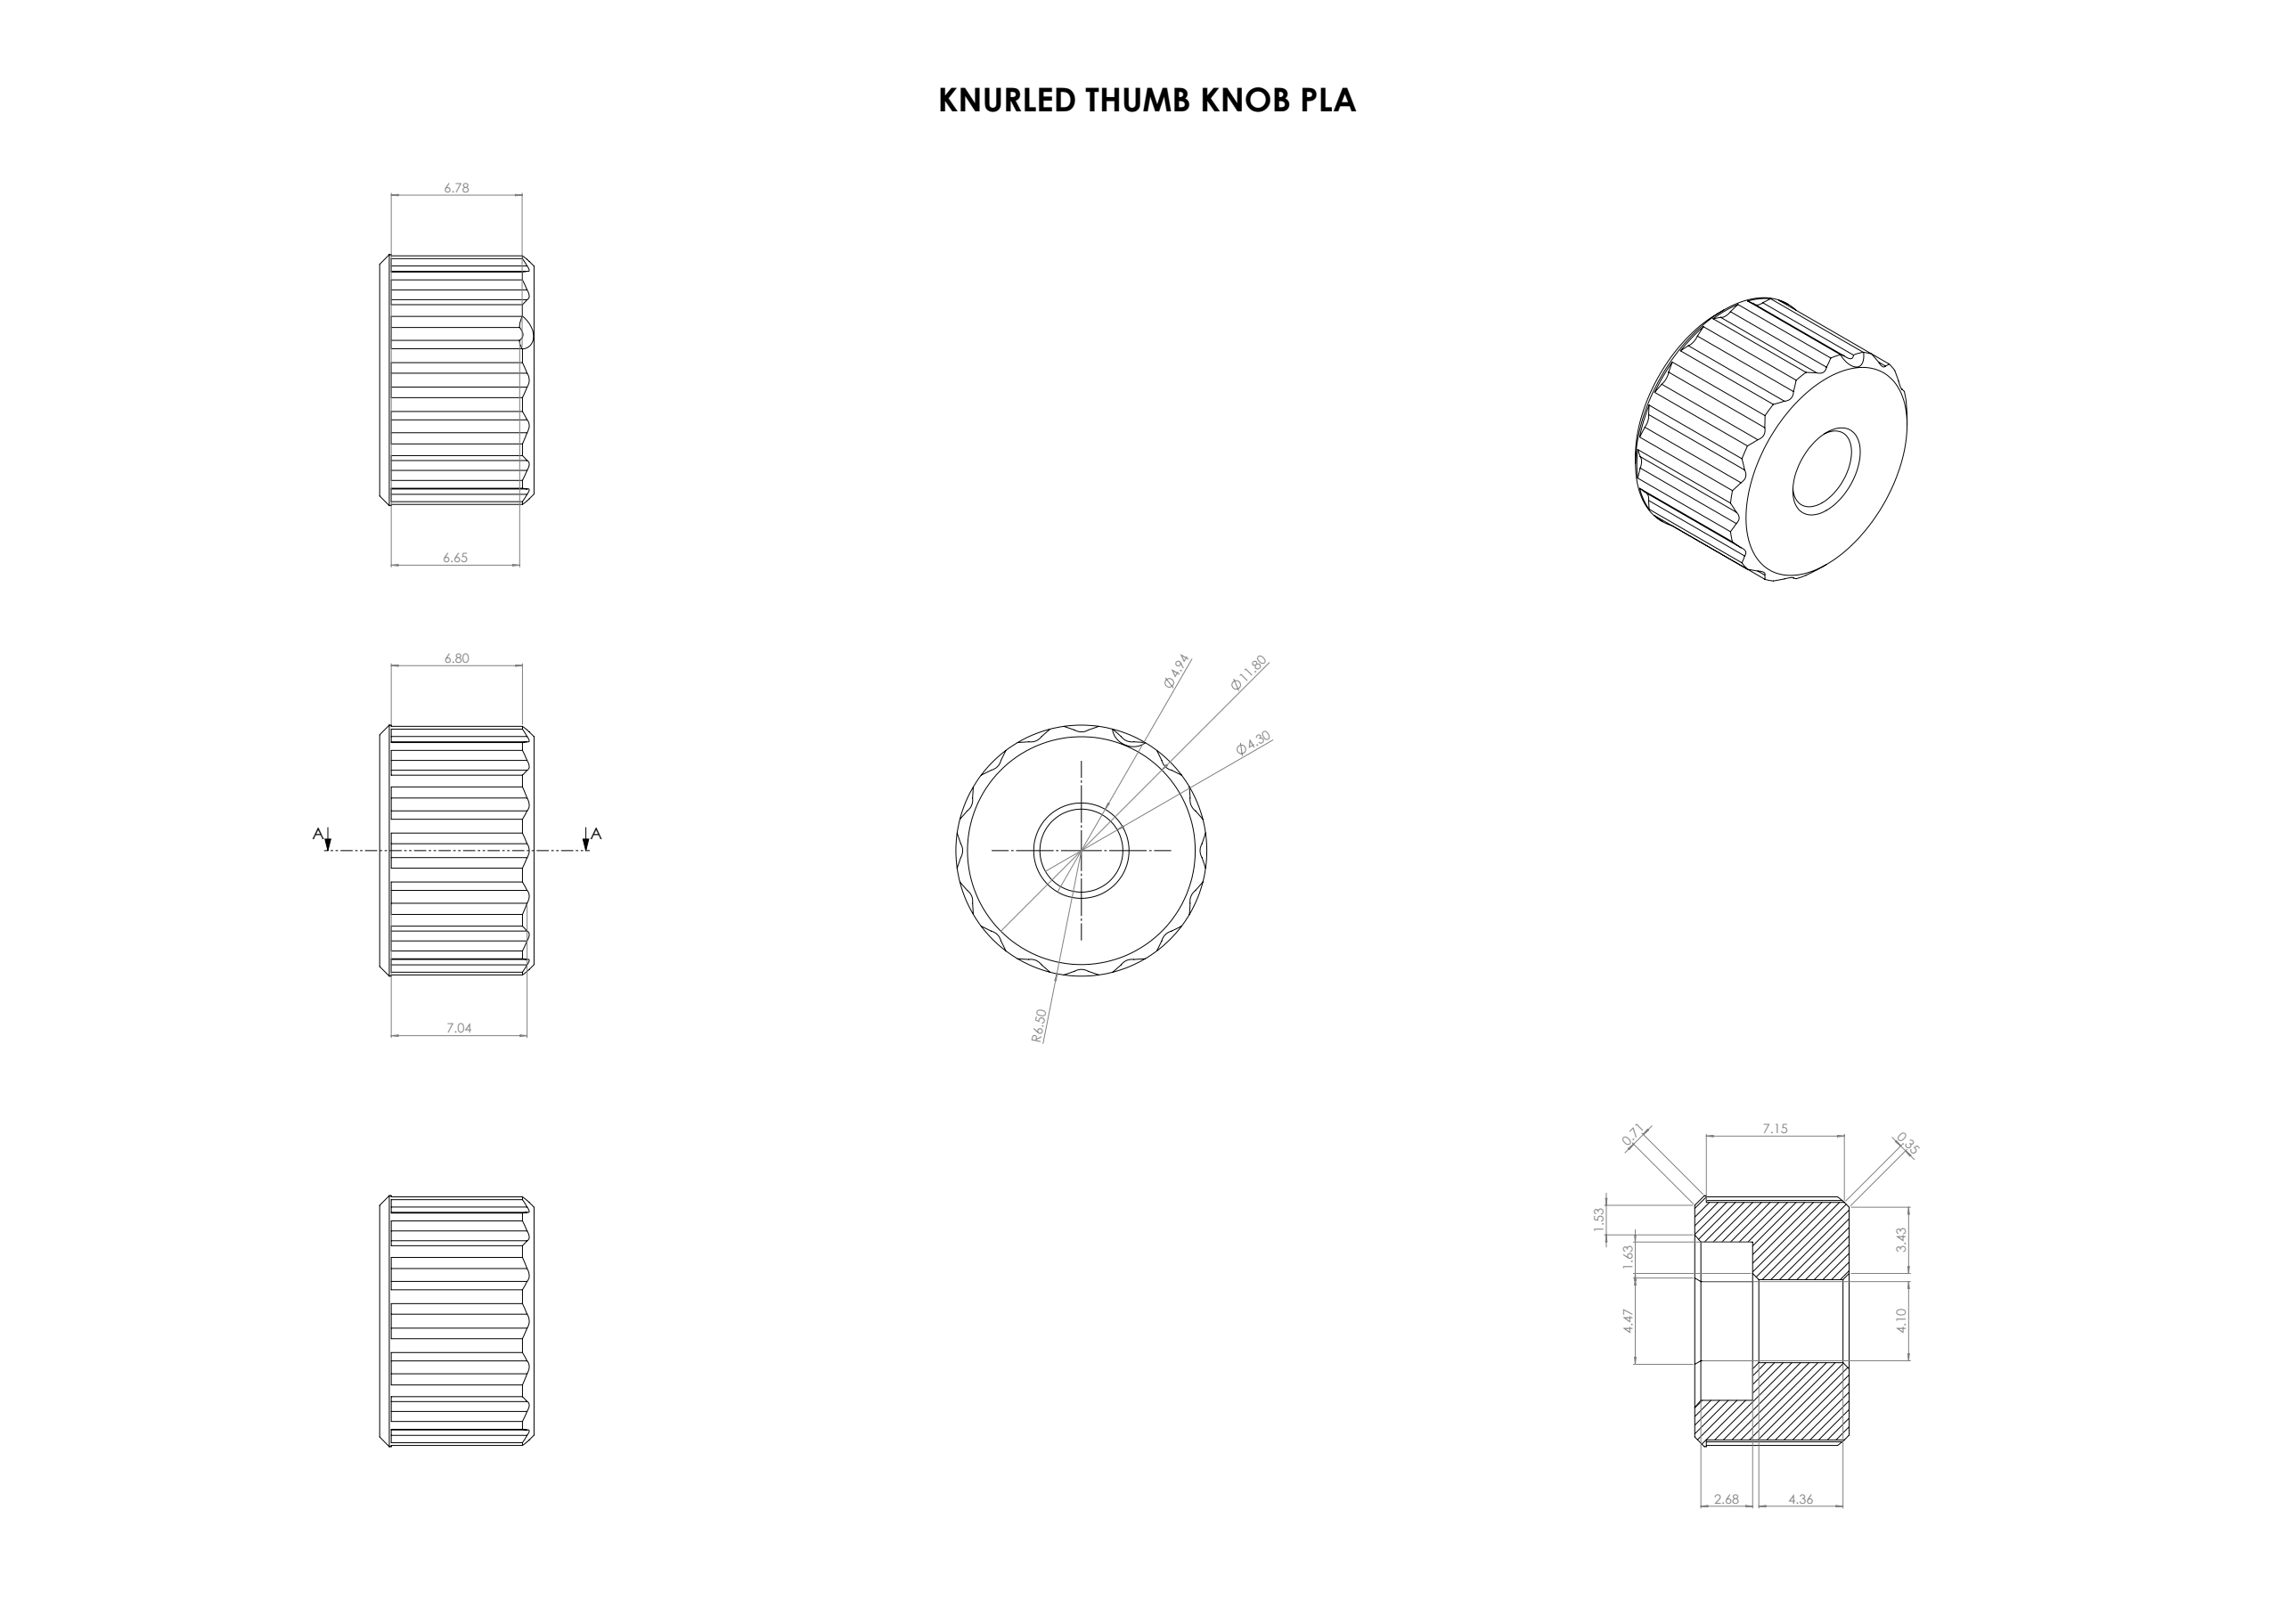
ISO-10303-21;
HEADER;
/* Generated by software containing ST-Developer
 * from STEP Tools, Inc. (www.steptools.com) 
 */

FILE_DESCRIPTION(
/* description */ (''),
/* implementation_level */ '2;1');

FILE_NAME(
/* name */ '08_Knurled_Thumb_Knob_PLA.step',
/* time_stamp */ '2026-10-21T02:01:14-07:00',
/* author */ (''),
/* organization */ (''),
/* preprocessor_version */ 'ST-DEVELOPER v20.2',
/* originating_system */ 'Autodesk Translation Framework v15.15.0.0',
/* authorisation */ '');

FILE_SCHEMA (('AUTOMOTIVE_DESIGN { 1 0 10303 214 3 1 1 }'));
ENDSEC;

DATA;
#10=MECHANICAL_DESIGN_GEOMETRIC_PRESENTATION_REPRESENTATION('',(#621),#37181);
#113=B_SPLINE_SURFACE_WITH_KNOTS('',3,3,((#26771,#26772,#26773,#26774,#26775,
#26776,#26777,#26778,#26779),(#26780,#26781,#26782,#26783,#26784,#26785,
#26786,#26787,#26788),(#26789,#26790,#26791,#26792,#26793,#26794,#26795,
#26796,#26797),(#26798,#26799,#26800,#26801,#26802,#26803,#26804,#26805,
#26806)),.UNSPECIFIED.,.F.,.F.,.F.,(4,4),(4,1,1,1,1,1,4),(0.,1.),(0.0342009647377285,
0.0587640238978664,0.0833270830580044,0.107890142218142,0.13245320137828,
0.181579319698556,0.206142378858694),.UNSPECIFIED.);
#259=B_SPLINE_CURVE_WITH_KNOTS('',3,(#26240,#26241,#26242,#26243),
 .UNSPECIFIED.,.F.,.F.,(4,4),(0.0531689808046697,0.0554215660138355),
 .UNSPECIFIED.);
#260=B_SPLINE_CURVE_WITH_KNOTS('',3,(#26251,#26252,#26253,#26254),
 .UNSPECIFIED.,.F.,.F.,(4,4),(0.,0.00224311679852086),.UNSPECIFIED.);
#261=B_SPLINE_CURVE_WITH_KNOTS('',3,(#26379,#26380,#26381,#26382,#26383,
#26384),.UNSPECIFIED.,.F.,.F.,(4,2,4),(0.120171671798206,0.144386237549695,
0.158573008898185),.UNSPECIFIED.);
#262=B_SPLINE_CURVE_WITH_KNOTS('',3,(#26393,#26394,#26395,#26396,#26397,
#26398,#26399,#26400,#26401,#26402),.UNSPECIFIED.,.F.,.F.,(4,2,2,2,4),(0.0817703346982273,
0.0959571060467179,0.120171671798206,0.144386237549695,0.158573008898185),
 .UNSPECIFIED.);
#263=B_SPLINE_CURVE_WITH_KNOTS('',3,(#26411,#26412,#26413,#26414,#26415,
#26416,#26417,#26418,#26419,#26420),.UNSPECIFIED.,.F.,.F.,(4,2,2,2,4),(0.0817703346982278,
0.095957106046718,0.120171671798206,0.144386237549695,0.158573008898185),
 .UNSPECIFIED.);
#264=B_SPLINE_CURVE_WITH_KNOTS('',3,(#26429,#26430,#26431,#26432,#26433,
#26434,#26435,#26436,#26437,#26438),.UNSPECIFIED.,.F.,.F.,(4,2,2,2,4),(0.0817703346982272,
0.0959571060467179,0.120171671798206,0.144386237549695,0.158573008898185),
 .UNSPECIFIED.);
#265=B_SPLINE_CURVE_WITH_KNOTS('',3,(#26447,#26448,#26449,#26450,#26451,
#26452,#26453,#26454,#26455,#26456),.UNSPECIFIED.,.F.,.F.,(4,2,2,2,4),(0.0817703346982273,
0.0959571060467178,0.120171671798206,0.144386237549695,0.158573008898185),
 .UNSPECIFIED.);
#266=B_SPLINE_CURVE_WITH_KNOTS('',3,(#26465,#26466,#26467,#26468,#26469,
#26470,#26471,#26472,#26473,#26474),.UNSPECIFIED.,.F.,.F.,(4,2,2,2,4),(0.081770334698227,
0.0959571060467179,0.120171671798206,0.144386237549695,0.158573008898185),
 .UNSPECIFIED.);
#267=B_SPLINE_CURVE_WITH_KNOTS('',3,(#26483,#26484,#26485,#26486,#26487,
#26488,#26489,#26490,#26491,#26492),.UNSPECIFIED.,.F.,.F.,(4,2,2,2,4),(0.0817703346982273,
0.0959571060467179,0.120171671798206,0.144386237549695,0.158573008898185),
 .UNSPECIFIED.);
#268=B_SPLINE_CURVE_WITH_KNOTS('',3,(#26496,#26497,#26498,#26499,#26500,
#26501,#26502,#26503,#26504),.UNSPECIFIED.,.F.,.F.,(4,1,1,1,1,1,4),(-0.20552137705515,
-0.181579319698556,-0.13245320137828,-0.107890142218142,-0.0833270830580044,
-0.0587640238978664,-0.0348207934698036),.UNSPECIFIED.);
#269=B_SPLINE_CURVE_WITH_KNOTS('',3,(#26506,#26507,#26508,#26509,#26510,
#26511,#26512,#26513,#26514,#26515),.UNSPECIFIED.,.F.,.F.,(4,2,2,2,4),(0.0817703346982273,
0.0959571060467179,0.120171671798206,0.144386237549695,0.158573008898185),
 .UNSPECIFIED.);
#270=B_SPLINE_CURVE_WITH_KNOTS('',3,(#26524,#26525,#26526,#26527,#26528,
#26529,#26530,#26531,#26532,#26533),.UNSPECIFIED.,.F.,.F.,(4,2,2,2,4),(0.0817703346982272,
0.095957106046718,0.120171671798206,0.144386237549695,0.158573008898185),
 .UNSPECIFIED.);
#271=B_SPLINE_CURVE_WITH_KNOTS('',3,(#26542,#26543,#26544,#26545,#26546,
#26547,#26548,#26549,#26550,#26551),.UNSPECIFIED.,.F.,.F.,(4,2,2,2,4),(0.0817703346982275,
0.095957106046718,0.120171671798206,0.144386237549695,0.158573008898185),
 .UNSPECIFIED.);
#272=B_SPLINE_CURVE_WITH_KNOTS('',3,(#26560,#26561,#26562,#26563,#26564,
#26565,#26566,#26567,#26568,#26569),.UNSPECIFIED.,.F.,.F.,(4,2,2,2,4),(0.0817703346982276,
0.095957106046718,0.120171671798206,0.144386237549695,0.158573008898185),
 .UNSPECIFIED.);
#273=B_SPLINE_CURVE_WITH_KNOTS('',3,(#26578,#26579,#26580,#26581,#26582,
#26583,#26584,#26585,#26586,#26587),.UNSPECIFIED.,.F.,.F.,(4,2,2,2,4),(0.0817703346982272,
0.0959571060467178,0.120171671798206,0.144386237549695,0.158573008898185),
 .UNSPECIFIED.);
#274=B_SPLINE_CURVE_WITH_KNOTS('',3,(#26596,#26597,#26598,#26599,#26600,
#26601,#26602,#26603,#26604,#26605),.UNSPECIFIED.,.F.,.F.,(4,2,2,2,4),(0.0817703346982273,
0.0959571060467179,0.120171671798206,0.144386237549695,0.158573008898185),
 .UNSPECIFIED.);
#275=B_SPLINE_CURVE_WITH_KNOTS('',3,(#26614,#26615,#26616,#26617,#26618,
#26619,#26620,#26621,#26622,#26623),.UNSPECIFIED.,.F.,.F.,(4,2,2,2,4),(0.0817703346982272,
0.0959571060467179,0.120171671798206,0.144386237549695,0.158573008898185),
 .UNSPECIFIED.);
#276=B_SPLINE_CURVE_WITH_KNOTS('',3,(#26632,#26633,#26634,#26635,#26636,
#26637,#26638,#26639,#26640,#26641),.UNSPECIFIED.,.F.,.F.,(4,2,2,2,4),(0.0817703346982276,
0.095957106046718,0.120171671798206,0.144386237549695,0.158573008898185),
 .UNSPECIFIED.);
#277=B_SPLINE_CURVE_WITH_KNOTS('',3,(#26649,#26650,#26651,#26652,#26653,
#26654),.UNSPECIFIED.,.F.,.F.,(4,2,4),(0.0817703346982272,0.0959571060467178,
0.120171671798206),.UNSPECIFIED.);
#278=B_SPLINE_CURVE_WITH_KNOTS('',3,(#26809,#26810,#26811,#26812,#26813,
#26814,#26815,#26816,#26817),.UNSPECIFIED.,.F.,.F.,(4,1,1,1,1,1,4),(0.0581066990795184,
0.0587640238978664,0.0833270830580044,0.107890142218142,0.13245320137828,
0.181579319698556,0.182236644516894),.UNSPECIFIED.);
#279=B_SPLINE_CURVE_WITH_KNOTS('',3,(#26818,#26819,#26820,#26821,#26822,
#26823,#26824,#26825),.UNSPECIFIED.,.F.,.F.,(4,2,2,4),(0.,0.0126311894885661,
0.032486538769803,0.052794817339328),.UNSPECIFIED.);
#280=B_SPLINE_CURVE_WITH_KNOTS('',3,(#26826,#26827,#26828,#26829,#26830,
#26831,#26832,#26833,#26834,#26835,#26836,#26837,#26838,#26839,#26840,#26841,
#26842,#26843,#26844,#26845,#26846,#26847,#26848,#26849,#26850),
 .UNSPECIFIED.,.F.,.F.,(4,3,3,3,3,3,3,3,4),(0.,0.011920157067792,0.0235023431475078,
0.0268086068446529,0.0354226971140202,0.0406217026705462,0.0495092313150064,
0.0577137413084294,0.0614436123664036),.UNSPECIFIED.);
#595=SHAPE_REPRESENTATION_RELATIONSHIP('SRR','None',#37245,#608);
#608=ADVANCED_BREP_SHAPE_REPRESENTATION('',(#634),#37175);
#621=STYLED_ITEM('',(#37387),#634);
#634=MANIFOLD_SOLID_BREP('Body1',#14783);
#678=FACE_BOUND('',#2790,.T.);
#679=FACE_BOUND('',#2829,.T.);
#680=FACE_BOUND('',#2840,.T.);
#786=CYLINDRICAL_SURFACE('',#15710,2.15);
#787=CYLINDRICAL_SURFACE('',#15715,6.5);
#788=CYLINDRICAL_SURFACE('',#15782,0.7);
#789=CYLINDRICAL_SURFACE('',#15802,0.7);
#790=CYLINDRICAL_SURFACE('',#15807,0.7);
#791=CYLINDRICAL_SURFACE('',#15808,0.7);
#792=CYLINDRICAL_SURFACE('',#15813,0.7);
#793=CYLINDRICAL_SURFACE('',#15814,0.7);
#794=CYLINDRICAL_SURFACE('',#15819,0.7);
#795=CYLINDRICAL_SURFACE('',#15820,0.7);
#796=CYLINDRICAL_SURFACE('',#15825,0.7);
#797=CYLINDRICAL_SURFACE('',#15826,0.7);
#798=CYLINDRICAL_SURFACE('',#15831,0.7);
#799=CYLINDRICAL_SURFACE('',#15832,0.7);
#800=CYLINDRICAL_SURFACE('',#15837,0.7);
#801=CYLINDRICAL_SURFACE('',#15838,0.7);
#802=CYLINDRICAL_SURFACE('',#15843,0.7);
#803=CYLINDRICAL_SURFACE('',#15844,0.7);
#1182=CIRCLE('',#15707,2.15);
#1183=CIRCLE('',#15708,2.15);
#1184=CIRCLE('',#15709,2.47);
#1185=CIRCLE('',#15711,2.15);
#1186=CIRCLE('',#15713,5.9);
#1187=CIRCLE('',#15716,6.5);
#1188=CIRCLE('',#15717,6.5);
#1189=CIRCLE('',#15718,6.5);
#1190=CIRCLE('',#15719,6.5);
#1191=CIRCLE('',#15720,6.5);
#1192=CIRCLE('',#15721,6.5);
#1193=CIRCLE('',#15722,6.5);
#1194=CIRCLE('',#15723,6.5);
#1195=CIRCLE('',#15724,6.5);
#1196=CIRCLE('',#15725,6.5);
#1197=CIRCLE('',#15726,6.5);
#1198=CIRCLE('',#15727,6.5);
#1199=CIRCLE('',#15728,6.5);
#1200=CIRCLE('',#15729,6.5);
#1201=CIRCLE('',#15730,6.5);
#1202=CIRCLE('',#15731,6.5);
#1203=CIRCLE('',#15732,6.5);
#1204=CIRCLE('',#15733,6.5);
#1205=CIRCLE('',#15734,6.5);
#1206=CIRCLE('',#15735,6.5);
#1207=CIRCLE('',#15736,6.5);
#1208=CIRCLE('',#15737,6.5);
#1209=CIRCLE('',#15738,6.5);
#1210=CIRCLE('',#15739,6.5);
#1211=CIRCLE('',#15740,6.5);
#1212=CIRCLE('',#15741,6.5);
#1213=CIRCLE('',#15742,6.5);
#1214=CIRCLE('',#15743,6.5);
#1215=CIRCLE('',#15744,6.5);
#1216=CIRCLE('',#15745,6.5);
#1217=CIRCLE('',#15746,6.5);
#1218=CIRCLE('',#15747,6.5);
#1219=CIRCLE('',#15748,6.5);
#1220=CIRCLE('',#15749,6.5);
#1221=CIRCLE('',#15783,0.7);
#1222=CIRCLE('',#15785,2.47);
#1223=CIRCLE('',#15797,6.);
#1224=CIRCLE('',#15803,0.7);
#1225=CIRCLE('',#15806,0.7);
#1226=CIRCLE('',#15809,0.7);
#1227=CIRCLE('',#15812,0.7);
#1228=CIRCLE('',#15815,0.7);
#1229=CIRCLE('',#15818,0.7);
#1230=CIRCLE('',#15821,0.7);
#1231=CIRCLE('',#15824,0.7);
#1232=CIRCLE('',#15827,0.7);
#1233=CIRCLE('',#15830,0.7);
#1234=CIRCLE('',#15833,0.7);
#1235=CIRCLE('',#15836,0.7);
#1236=CIRCLE('',#15839,0.7);
#1237=CIRCLE('',#15842,0.7);
#1238=CIRCLE('',#15845,0.7);
#1352=CONICAL_SURFACE('',#15706,2.31,0.785398163397448);
#1353=CONICAL_SURFACE('',#15750,6.2,0.785398163397447);
#1354=CONICAL_SURFACE('',#15784,2.31,0.785398163397448);
#1355=CONICAL_SURFACE('',#15847,6.25,0.785398163397449);
#1909=FACE_OUTER_BOUND('',#2787,.T.);
#1910=FACE_OUTER_BOUND('',#2788,.T.);
#1911=FACE_OUTER_BOUND('',#2789,.T.);
#1912=FACE_OUTER_BOUND('',#2791,.T.);
#1913=FACE_OUTER_BOUND('',#2792,.T.);
#1914=FACE_OUTER_BOUND('',#2793,.T.);
#1915=FACE_OUTER_BOUND('',#2794,.T.);
#1916=FACE_OUTER_BOUND('',#2795,.T.);
#1917=FACE_OUTER_BOUND('',#2796,.T.);
#1918=FACE_OUTER_BOUND('',#2797,.T.);
#1919=FACE_OUTER_BOUND('',#2798,.T.);
#1920=FACE_OUTER_BOUND('',#2799,.T.);
#1921=FACE_OUTER_BOUND('',#2800,.T.);
#1922=FACE_OUTER_BOUND('',#2801,.T.);
#1923=FACE_OUTER_BOUND('',#2802,.T.);
#1924=FACE_OUTER_BOUND('',#2803,.T.);
#1925=FACE_OUTER_BOUND('',#2804,.T.);
#1926=FACE_OUTER_BOUND('',#2805,.T.);
#1927=FACE_OUTER_BOUND('',#2806,.T.);
#1928=FACE_OUTER_BOUND('',#2807,.T.);
#1929=FACE_OUTER_BOUND('',#2808,.T.);
#1930=FACE_OUTER_BOUND('',#2809,.T.);
#1931=FACE_OUTER_BOUND('',#2810,.T.);
#1932=FACE_OUTER_BOUND('',#2811,.T.);
#1933=FACE_OUTER_BOUND('',#2812,.T.);
#1934=FACE_OUTER_BOUND('',#2813,.T.);
#1935=FACE_OUTER_BOUND('',#2814,.T.);
#1936=FACE_OUTER_BOUND('',#2815,.T.);
#1937=FACE_OUTER_BOUND('',#2816,.T.);
#1938=FACE_OUTER_BOUND('',#2817,.T.);
#1939=FACE_OUTER_BOUND('',#2818,.T.);
#1940=FACE_OUTER_BOUND('',#2819,.T.);
#1941=FACE_OUTER_BOUND('',#2820,.T.);
#1942=FACE_OUTER_BOUND('',#2821,.T.);
#1943=FACE_OUTER_BOUND('',#2822,.T.);
#1944=FACE_OUTER_BOUND('',#2823,.T.);
#1945=FACE_OUTER_BOUND('',#2824,.T.);
#1946=FACE_OUTER_BOUND('',#2825,.T.);
#1947=FACE_OUTER_BOUND('',#2826,.T.);
#1948=FACE_OUTER_BOUND('',#2827,.T.);
#1949=FACE_OUTER_BOUND('',#2828,.T.);
#1950=FACE_OUTER_BOUND('',#2830,.T.);
#1951=FACE_OUTER_BOUND('',#2831,.T.);
#1952=FACE_OUTER_BOUND('',#2832,.T.);
#1953=FACE_OUTER_BOUND('',#2833,.T.);
#1954=FACE_OUTER_BOUND('',#2834,.T.);
#1955=FACE_OUTER_BOUND('',#2835,.T.);
#1956=FACE_OUTER_BOUND('',#2836,.T.);
#1957=FACE_OUTER_BOUND('',#2837,.T.);
#1958=FACE_OUTER_BOUND('',#2838,.T.);
#1959=FACE_OUTER_BOUND('',#2839,.T.);
#1960=FACE_OUTER_BOUND('',#2841,.T.);
#1961=FACE_OUTER_BOUND('',#2842,.T.);
#1962=FACE_OUTER_BOUND('',#2843,.T.);
#1963=FACE_OUTER_BOUND('',#2844,.T.);
#1964=FACE_OUTER_BOUND('',#2845,.T.);
#1965=FACE_OUTER_BOUND('',#2846,.T.);
#1966=FACE_OUTER_BOUND('',#2847,.T.);
#1967=FACE_OUTER_BOUND('',#2848,.T.);
#1968=FACE_OUTER_BOUND('',#2849,.T.);
#1969=FACE_OUTER_BOUND('',#2850,.T.);
#1970=FACE_OUTER_BOUND('',#2851,.T.);
#1971=FACE_OUTER_BOUND('',#2852,.T.);
#1972=FACE_OUTER_BOUND('',#2853,.T.);
#1973=FACE_OUTER_BOUND('',#2854,.T.);
#1974=FACE_OUTER_BOUND('',#2855,.T.);
#1975=FACE_OUTER_BOUND('',#2856,.T.);
#1976=FACE_OUTER_BOUND('',#2857,.T.);
#1977=FACE_OUTER_BOUND('',#2858,.T.);
#1978=FACE_OUTER_BOUND('',#2859,.T.);
#1979=FACE_OUTER_BOUND('',#2860,.T.);
#1980=FACE_OUTER_BOUND('',#2861,.T.);
#1981=FACE_OUTER_BOUND('',#2862,.T.);
#1982=FACE_OUTER_BOUND('',#2863,.T.);
#1983=FACE_OUTER_BOUND('',#2864,.T.);
#1984=FACE_OUTER_BOUND('',#2865,.T.);
#1985=FACE_OUTER_BOUND('',#2866,.T.);
#1986=FACE_OUTER_BOUND('',#2867,.T.);
#1987=FACE_OUTER_BOUND('',#2868,.T.);
#1988=FACE_OUTER_BOUND('',#2869,.T.);
#1989=FACE_OUTER_BOUND('',#2870,.T.);
#1990=FACE_OUTER_BOUND('',#2871,.T.);
#1991=FACE_OUTER_BOUND('',#2872,.T.);
#1992=FACE_OUTER_BOUND('',#2873,.T.);
#1993=FACE_OUTER_BOUND('',#2874,.T.);
#1994=FACE_OUTER_BOUND('',#2875,.T.);
#2787=EDGE_LOOP('',(#11803,#11804,#11805,#11806,#11807));
#2788=EDGE_LOOP('',(#11808,#11809,#11810,#11811,#11812));
#2789=EDGE_LOOP('',(#11813));
#2790=EDGE_LOOP('',(#11814));
#2791=EDGE_LOOP('',(#11815,#11816,#11817,#11818));
#2792=EDGE_LOOP('',(#11819,#11820,#11821,#11822,#11823,#11824,#11825,#11826,
#11827,#11828,#11829,#11830,#11831,#11832,#11833,#11834,#11835,#11836,#11837,
#11838,#11839,#11840,#11841,#11842,#11843,#11844,#11845,#11846,#11847,#11848,
#11849,#11850,#11851,#11852,#11853,#11854,#11855,#11856,#11857,#11858,#11859,
#11860,#11861,#11862,#11863,#11864,#11865,#11866,#11867,#11868,#11869,#11870,
#11871,#11872,#11873,#11874,#11875,#11876,#11877,#11878,#11879,#11880,#11881,
#11882,#11883,#11884,#11885,#11886,#11887,#11888));
#2793=EDGE_LOOP('',(#11889,#11890,#11891,#11892,#11893,#11894,#11895,#11896,
#11897,#11898,#11899,#11900,#11901,#11902,#11903,#11904,#11905,#11906,#11907,
#11908,#11909,#11910,#11911,#11912,#11913,#11914,#11915,#11916,#11917,#11918,
#11919,#11920,#11921,#11922,#11923,#11924,#11925,#11926,#11927,#11928,#11929,
#11930,#11931,#11932,#11933,#11934,#11935,#11936,#11937,#11938,#11939,#11940,
#11941,#11942,#11943,#11944,#11945,#11946,#11947,#11948,#11949,#11950,#11951,
#11952,#11953,#11954));
#2794=EDGE_LOOP('',(#11955,#11956,#11957,#11958));
#2795=EDGE_LOOP('',(#11959,#11960,#11961,#11962));
#2796=EDGE_LOOP('',(#11963,#11964,#11965,#11966));
#2797=EDGE_LOOP('',(#11967,#11968,#11969,#11970));
#2798=EDGE_LOOP('',(#11971,#11972,#11973,#11974));
#2799=EDGE_LOOP('',(#11975,#11976,#11977,#11978));
#2800=EDGE_LOOP('',(#11979,#11980,#11981,#11982));
#2801=EDGE_LOOP('',(#11983,#11984,#11985,#11986));
#2802=EDGE_LOOP('',(#11987,#11988,#11989,#11990));
#2803=EDGE_LOOP('',(#11991,#11992,#11993,#11994));
#2804=EDGE_LOOP('',(#11995,#11996,#11997,#11998));
#2805=EDGE_LOOP('',(#11999,#12000,#12001,#12002));
#2806=EDGE_LOOP('',(#12003,#12004,#12005,#12006));
#2807=EDGE_LOOP('',(#12007,#12008,#12009,#12010));
#2808=EDGE_LOOP('',(#12011,#12012,#12013,#12014));
#2809=EDGE_LOOP('',(#12015,#12016,#12017,#12018));
#2810=EDGE_LOOP('',(#12019,#12020,#12021,#12022));
#2811=EDGE_LOOP('',(#12023,#12024,#12025,#12026));
#2812=EDGE_LOOP('',(#12027,#12028,#12029,#12030));
#2813=EDGE_LOOP('',(#12031,#12032,#12033,#12034));
#2814=EDGE_LOOP('',(#12035,#12036,#12037,#12038));
#2815=EDGE_LOOP('',(#12039,#12040,#12041,#12042));
#2816=EDGE_LOOP('',(#12043,#12044,#12045,#12046));
#2817=EDGE_LOOP('',(#12047,#12048,#12049,#12050));
#2818=EDGE_LOOP('',(#12051,#12052,#12053,#12054));
#2819=EDGE_LOOP('',(#12055,#12056,#12057,#12058));
#2820=EDGE_LOOP('',(#12059,#12060,#12061,#12062));
#2821=EDGE_LOOP('',(#12063,#12064,#12065,#12066));
#2822=EDGE_LOOP('',(#12067,#12068,#12069,#12070));
#2823=EDGE_LOOP('',(#12071,#12072,#12073,#12074,#12075,#12076));
#2824=EDGE_LOOP('',(#12077,#12078,#12079,#12080));
#2825=EDGE_LOOP('',(#12081,#12082,#12083,#12084));
#2826=EDGE_LOOP('',(#12085,#12086,#12087,#12088));
#2827=EDGE_LOOP('',(#12089,#12090,#12091,#12092));
#2828=EDGE_LOOP('',(#12093,#12094,#12095,#12096,#12097,#12098));
#2829=EDGE_LOOP('',(#12099));
#2830=EDGE_LOOP('',(#12100,#12101,#12102,#12103));
#2831=EDGE_LOOP('',(#12104,#12105,#12106,#12107));
#2832=EDGE_LOOP('',(#12108,#12109,#12110,#12111));
#2833=EDGE_LOOP('',(#12112,#12113,#12114,#12115));
#2834=EDGE_LOOP('',(#12116,#12117,#12118,#12119));
#2835=EDGE_LOOP('',(#12120,#12121,#12122,#12123));
#2836=EDGE_LOOP('',(#12124,#12125,#12126,#12127));
#2837=EDGE_LOOP('',(#12128,#12129,#12130,#12131));
#2838=EDGE_LOOP('',(#12132,#12133,#12134,#12135));
#2839=EDGE_LOOP('',(#12136));
#2840=EDGE_LOOP('',(#12137,#12138,#12139,#12140,#12141,#12142));
#2841=EDGE_LOOP('',(#12143,#12144,#12145,#12146));
#2842=EDGE_LOOP('',(#12147,#12148,#12149,#12150));
#2843=EDGE_LOOP('',(#12151,#12152,#12153,#12154));
#2844=EDGE_LOOP('',(#12155,#12156,#12157,#12158));
#2845=EDGE_LOOP('',(#12159,#12160,#12161,#12162));
#2846=EDGE_LOOP('',(#12163,#12164,#12165,#12166));
#2847=EDGE_LOOP('',(#12167,#12168,#12169,#12170));
#2848=EDGE_LOOP('',(#12171,#12172,#12173,#12174));
#2849=EDGE_LOOP('',(#12175,#12176,#12177,#12178));
#2850=EDGE_LOOP('',(#12179,#12180,#12181,#12182));
#2851=EDGE_LOOP('',(#12183,#12184,#12185,#12186));
#2852=EDGE_LOOP('',(#12187,#12188,#12189,#12190));
#2853=EDGE_LOOP('',(#12191,#12192,#12193,#12194));
#2854=EDGE_LOOP('',(#12195,#12196,#12197,#12198));
#2855=EDGE_LOOP('',(#12199,#12200,#12201,#12202));
#2856=EDGE_LOOP('',(#12203,#12204,#12205,#12206));
#2857=EDGE_LOOP('',(#12207,#12208,#12209,#12210,#12211));
#2858=EDGE_LOOP('',(#12212,#12213,#12214,#12215,#12216));
#2859=EDGE_LOOP('',(#12217,#12218,#12219,#12220));
#2860=EDGE_LOOP('',(#12221,#12222,#12223,#12224));
#2861=EDGE_LOOP('',(#12225,#12226,#12227,#12228));
#2862=EDGE_LOOP('',(#12229,#12230,#12231,#12232));
#2863=EDGE_LOOP('',(#12233,#12234,#12235,#12236));
#2864=EDGE_LOOP('',(#12237,#12238,#12239,#12240));
#2865=EDGE_LOOP('',(#12241,#12242,#12243,#12244));
#2866=EDGE_LOOP('',(#12245,#12246,#12247,#12248));
#2867=EDGE_LOOP('',(#12249,#12250,#12251,#12252));
#2868=EDGE_LOOP('',(#12253,#12254,#12255,#12256));
#2869=EDGE_LOOP('',(#12257,#12258,#12259,#12260));
#2870=EDGE_LOOP('',(#12261,#12262,#12263,#12264));
#2871=EDGE_LOOP('',(#12265,#12266,#12267,#12268));
#2872=EDGE_LOOP('',(#12269,#12270,#12271,#12272));
#2873=EDGE_LOOP('',(#12273,#12274,#12275,#12276));
#2874=EDGE_LOOP('',(#12277,#12278,#12279,#12280));
#2875=EDGE_LOOP('',(#12281,#12282,#12283,#12284));
#3138=(
BOUNDED_CURVE()
B_SPLINE_CURVE(2,(#26226,#26227,#26228),.UNSPECIFIED.,.F.,.F.)
B_SPLINE_CURVE_WITH_KNOTS((3,3),(0.136653338911782,0.195398016960284),
 .UNSPECIFIED.)
CURVE()
GEOMETRIC_REPRESENTATION_ITEM()
RATIONAL_B_SPLINE_CURVE((1.00492385476096,1.00359200155149,1.00020515445013))
REPRESENTATION_ITEM('')
);
#3139=(
BOUNDED_CURVE()
B_SPLINE_CURVE(2,(#26385,#26386,#26387),.UNSPECIFIED.,.F.,.F.)
B_SPLINE_CURVE_WITH_KNOTS((3,3),(0.0017631420801792,0.0605078201286812),
 .UNSPECIFIED.)
CURVE()
GEOMETRIC_REPRESENTATION_ITEM()
RATIONAL_B_SPLINE_CURVE((1.00020515445013,1.00359200155149,1.00492385476096))
REPRESENTATION_ITEM('')
);
#3140=(
BOUNDED_CURVE()
B_SPLINE_CURVE(2,(#26389,#26390,#26391),.UNSPECIFIED.,.F.,.F.)
B_SPLINE_CURVE_WITH_KNOTS((3,3),(0.136653338911781,0.195398016960283),
 .UNSPECIFIED.)
CURVE()
GEOMETRIC_REPRESENTATION_ITEM()
RATIONAL_B_SPLINE_CURVE((1.00492385476097,1.0035920015515,1.00020515445013))
REPRESENTATION_ITEM('')
);
#3141=(
BOUNDED_CURVE()
B_SPLINE_CURVE(2,(#26403,#26404,#26405),.UNSPECIFIED.,.F.,.F.)
B_SPLINE_CURVE_WITH_KNOTS((3,3),(0.00176314208017943,0.060507820128681),
 .UNSPECIFIED.)
CURVE()
GEOMETRIC_REPRESENTATION_ITEM()
RATIONAL_B_SPLINE_CURVE((1.00020515445013,1.00359200155151,1.00492385476097))
REPRESENTATION_ITEM('')
);
#3142=(
BOUNDED_CURVE()
B_SPLINE_CURVE(2,(#26407,#26408,#26409),.UNSPECIFIED.,.F.,.F.)
B_SPLINE_CURVE_WITH_KNOTS((3,3),(0.136653338911775,0.195398016960278),
 .UNSPECIFIED.)
CURVE()
GEOMETRIC_REPRESENTATION_ITEM()
RATIONAL_B_SPLINE_CURVE((1.00492385476094,1.00359200155148,1.00020515445012))
REPRESENTATION_ITEM('')
);
#3143=(
BOUNDED_CURVE()
B_SPLINE_CURVE(2,(#26421,#26422,#26423),.UNSPECIFIED.,.F.,.F.)
B_SPLINE_CURVE_WITH_KNOTS((3,3),(0.00176314208017901,0.0605078201286807),
 .UNSPECIFIED.)
CURVE()
GEOMETRIC_REPRESENTATION_ITEM()
RATIONAL_B_SPLINE_CURVE((1.00020515445013,1.0035920015515,1.00492385476096))
REPRESENTATION_ITEM('')
);
#3144=(
BOUNDED_CURVE()
B_SPLINE_CURVE(2,(#26425,#26426,#26427),.UNSPECIFIED.,.F.,.F.)
B_SPLINE_CURVE_WITH_KNOTS((3,3),(0.136653338911781,0.195398016960283),
 .UNSPECIFIED.)
CURVE()
GEOMETRIC_REPRESENTATION_ITEM()
RATIONAL_B_SPLINE_CURVE((1.00492385476095,1.00359200155149,1.00020515445012))
REPRESENTATION_ITEM('')
);
#3145=(
BOUNDED_CURVE()
B_SPLINE_CURVE(2,(#26439,#26440,#26441),.UNSPECIFIED.,.F.,.F.)
B_SPLINE_CURVE_WITH_KNOTS((3,3),(0.00176314208017882,0.0605078201286799),
 .UNSPECIFIED.)
CURVE()
GEOMETRIC_REPRESENTATION_ITEM()
RATIONAL_B_SPLINE_CURVE((1.00020515445013,1.00359200155151,1.00492385476098))
REPRESENTATION_ITEM('')
);
#3146=(
BOUNDED_CURVE()
B_SPLINE_CURVE(2,(#26443,#26444,#26445),.UNSPECIFIED.,.F.,.F.)
B_SPLINE_CURVE_WITH_KNOTS((3,3),(0.136653338911781,0.195398016960283),
 .UNSPECIFIED.)
CURVE()
GEOMETRIC_REPRESENTATION_ITEM()
RATIONAL_B_SPLINE_CURVE((1.00492385476096,1.0035920015515,1.00020515445013))
REPRESENTATION_ITEM('')
);
#3147=(
BOUNDED_CURVE()
B_SPLINE_CURVE(2,(#26457,#26458,#26459),.UNSPECIFIED.,.F.,.F.)
B_SPLINE_CURVE_WITH_KNOTS((3,3),(0.0017631420801791,0.0605078201286811),
 .UNSPECIFIED.)
CURVE()
GEOMETRIC_REPRESENTATION_ITEM()
RATIONAL_B_SPLINE_CURVE((1.00020515445012,1.00359200155149,1.00492385476095))
REPRESENTATION_ITEM('')
);
#3148=(
BOUNDED_CURVE()
B_SPLINE_CURVE(2,(#26461,#26462,#26463),.UNSPECIFIED.,.F.,.F.)
B_SPLINE_CURVE_WITH_KNOTS((3,3),(0.136653338911783,0.195398016960284),
 .UNSPECIFIED.)
CURVE()
GEOMETRIC_REPRESENTATION_ITEM()
RATIONAL_B_SPLINE_CURVE((1.00492385476097,1.0035920015515,1.00020515445013))
REPRESENTATION_ITEM('')
);
#3149=(
BOUNDED_CURVE()
B_SPLINE_CURVE(2,(#26475,#26476,#26477),.UNSPECIFIED.,.F.,.F.)
B_SPLINE_CURVE_WITH_KNOTS((3,3),(0.00176314208017924,0.0605078201286807),
 .UNSPECIFIED.)
CURVE()
GEOMETRIC_REPRESENTATION_ITEM()
RATIONAL_B_SPLINE_CURVE((1.00020515445013,1.00359200155151,1.00492385476097))
REPRESENTATION_ITEM('')
);
#3150=(
BOUNDED_CURVE()
B_SPLINE_CURVE(2,(#26479,#26480,#26481),.UNSPECIFIED.,.F.,.F.)
B_SPLINE_CURVE_WITH_KNOTS((3,3),(0.136653338911782,0.195398016960284),
 .UNSPECIFIED.)
CURVE()
GEOMETRIC_REPRESENTATION_ITEM()
RATIONAL_B_SPLINE_CURVE((1.00492385476095,1.00359200155149,1.00020515445012))
REPRESENTATION_ITEM('')
);
#3151=(
BOUNDED_CURVE()
B_SPLINE_CURVE(2,(#26493,#26494,#26495),.UNSPECIFIED.,.F.,.F.)
B_SPLINE_CURVE_WITH_KNOTS((3,3),(0.00176314208017894,0.06050782012868),
 .UNSPECIFIED.)
CURVE()
GEOMETRIC_REPRESENTATION_ITEM()
RATIONAL_B_SPLINE_CURVE((1.00020515445013,1.00359200155151,1.00492385476098))
REPRESENTATION_ITEM('')
);
#3152=(
BOUNDED_CURVE()
B_SPLINE_CURVE(2,(#26516,#26517,#26518),.UNSPECIFIED.,.F.,.F.)
B_SPLINE_CURVE_WITH_KNOTS((3,3),(0.00176314208017899,0.0605078201286809),
 .UNSPECIFIED.)
CURVE()
GEOMETRIC_REPRESENTATION_ITEM()
RATIONAL_B_SPLINE_CURVE((1.00020515445012,1.00359200155149,1.00492385476096))
REPRESENTATION_ITEM('')
);
#3153=(
BOUNDED_CURVE()
B_SPLINE_CURVE(2,(#26520,#26521,#26522),.UNSPECIFIED.,.F.,.F.)
B_SPLINE_CURVE_WITH_KNOTS((3,3),(0.136653338911781,0.195398016960282),
 .UNSPECIFIED.)
CURVE()
GEOMETRIC_REPRESENTATION_ITEM()
RATIONAL_B_SPLINE_CURVE((1.00492385476097,1.0035920015515,1.00020515445013))
REPRESENTATION_ITEM('')
);
#3154=(
BOUNDED_CURVE()
B_SPLINE_CURVE(2,(#26534,#26535,#26536),.UNSPECIFIED.,.F.,.F.)
B_SPLINE_CURVE_WITH_KNOTS((3,3),(0.00176314208017926,0.0605078201286816),
 .UNSPECIFIED.)
CURVE()
GEOMETRIC_REPRESENTATION_ITEM()
RATIONAL_B_SPLINE_CURVE((1.00020515445013,1.00359200155149,1.00492385476096))
REPRESENTATION_ITEM('')
);
#3155=(
BOUNDED_CURVE()
B_SPLINE_CURVE(2,(#26538,#26539,#26540),.UNSPECIFIED.,.F.,.F.)
B_SPLINE_CURVE_WITH_KNOTS((3,3),(0.136653338911783,0.195398016960284),
 .UNSPECIFIED.)
CURVE()
GEOMETRIC_REPRESENTATION_ITEM()
RATIONAL_B_SPLINE_CURVE((1.00492385476097,1.00359200155151,1.00020515445013))
REPRESENTATION_ITEM('')
);
#3156=(
BOUNDED_CURVE()
B_SPLINE_CURVE(2,(#26552,#26553,#26554),.UNSPECIFIED.,.F.,.F.)
B_SPLINE_CURVE_WITH_KNOTS((3,3),(0.00176314208017907,0.0605078201286811),
 .UNSPECIFIED.)
CURVE()
GEOMETRIC_REPRESENTATION_ITEM()
RATIONAL_B_SPLINE_CURVE((1.00020515445012,1.00359200155149,1.00492385476096))
REPRESENTATION_ITEM('')
);
#3157=(
BOUNDED_CURVE()
B_SPLINE_CURVE(2,(#26556,#26557,#26558),.UNSPECIFIED.,.F.,.F.)
B_SPLINE_CURVE_WITH_KNOTS((3,3),(0.136653338911777,0.19539801696028),
 .UNSPECIFIED.)
CURVE()
GEOMETRIC_REPRESENTATION_ITEM()
RATIONAL_B_SPLINE_CURVE((1.00492385476094,1.00359200155149,1.00020515445012))
REPRESENTATION_ITEM('')
);
#3158=(
BOUNDED_CURVE()
B_SPLINE_CURVE(2,(#26570,#26571,#26572),.UNSPECIFIED.,.F.,.F.)
B_SPLINE_CURVE_WITH_KNOTS((3,3),(0.00176314208017916,0.0605078201286813),
 .UNSPECIFIED.)
CURVE()
GEOMETRIC_REPRESENTATION_ITEM()
RATIONAL_B_SPLINE_CURVE((1.00020515445012,1.00359200155149,1.00492385476095))
REPRESENTATION_ITEM('')
);
#3159=(
BOUNDED_CURVE()
B_SPLINE_CURVE(2,(#26574,#26575,#26576),.UNSPECIFIED.,.F.,.F.)
B_SPLINE_CURVE_WITH_KNOTS((3,3),(0.136653338911781,0.195398016960283),
 .UNSPECIFIED.)
CURVE()
GEOMETRIC_REPRESENTATION_ITEM()
RATIONAL_B_SPLINE_CURVE((1.00492385476096,1.0035920015515,1.00020515445013))
REPRESENTATION_ITEM('')
);
#3160=(
BOUNDED_CURVE()
B_SPLINE_CURVE(2,(#26588,#26589,#26590),.UNSPECIFIED.,.F.,.F.)
B_SPLINE_CURVE_WITH_KNOTS((3,3),(0.00176314208017902,0.060507820128681),
 .UNSPECIFIED.)
CURVE()
GEOMETRIC_REPRESENTATION_ITEM()
RATIONAL_B_SPLINE_CURVE((1.00020515445012,1.00359200155149,1.00492385476096))
REPRESENTATION_ITEM('')
);
#3161=(
BOUNDED_CURVE()
B_SPLINE_CURVE(2,(#26592,#26593,#26594),.UNSPECIFIED.,.F.,.F.)
B_SPLINE_CURVE_WITH_KNOTS((3,3),(0.13665333891178,0.195398016960282),
 .UNSPECIFIED.)
CURVE()
GEOMETRIC_REPRESENTATION_ITEM()
RATIONAL_B_SPLINE_CURVE((1.00492385476095,1.00359200155149,1.00020515445012))
REPRESENTATION_ITEM('')
);
#3162=(
BOUNDED_CURVE()
B_SPLINE_CURVE(2,(#26606,#26607,#26608),.UNSPECIFIED.,.F.,.F.)
B_SPLINE_CURVE_WITH_KNOTS((3,3),(0.00176314208017895,0.0605078201286814),
 .UNSPECIFIED.)
CURVE()
GEOMETRIC_REPRESENTATION_ITEM()
RATIONAL_B_SPLINE_CURVE((1.00020515445012,1.00359200155149,1.00492385476095))
REPRESENTATION_ITEM('')
);
#3163=(
BOUNDED_CURVE()
B_SPLINE_CURVE(2,(#26610,#26611,#26612),.UNSPECIFIED.,.F.,.F.)
B_SPLINE_CURVE_WITH_KNOTS((3,3),(0.136653338911781,0.195398016960283),
 .UNSPECIFIED.)
CURVE()
GEOMETRIC_REPRESENTATION_ITEM()
RATIONAL_B_SPLINE_CURVE((1.00492385476096,1.00359200155149,1.00020515445012))
REPRESENTATION_ITEM('')
);
#3164=(
BOUNDED_CURVE()
B_SPLINE_CURVE(2,(#26624,#26625,#26626),.UNSPECIFIED.,.F.,.F.)
B_SPLINE_CURVE_WITH_KNOTS((3,3),(0.00176314208017911,0.0605078201286809),
 .UNSPECIFIED.)
CURVE()
GEOMETRIC_REPRESENTATION_ITEM()
RATIONAL_B_SPLINE_CURVE((1.00020515445013,1.0035920015515,1.00492385476096))
REPRESENTATION_ITEM('')
);
#3165=(
BOUNDED_CURVE()
B_SPLINE_CURVE(2,(#26628,#26629,#26630),.UNSPECIFIED.,.F.,.F.)
B_SPLINE_CURVE_WITH_KNOTS((3,3),(0.136653338911778,0.19539801696028),
 .UNSPECIFIED.)
CURVE()
GEOMETRIC_REPRESENTATION_ITEM()
RATIONAL_B_SPLINE_CURVE((1.00492385476096,1.0035920015515,1.00020515445013))
REPRESENTATION_ITEM('')
);
#3166=(
BOUNDED_CURVE()
B_SPLINE_CURVE(2,(#26642,#26643,#26644),.UNSPECIFIED.,.F.,.F.)
B_SPLINE_CURVE_WITH_KNOTS((3,3),(0.00176314208017945,0.0605078201286828),
 .UNSPECIFIED.)
CURVE()
GEOMETRIC_REPRESENTATION_ITEM()
RATIONAL_B_SPLINE_CURVE((1.00020515445012,1.00359200155148,1.00492385476094))
REPRESENTATION_ITEM('')
);
#3167=(
BOUNDED_CURVE()
B_SPLINE_CURVE(2,(#26646,#26647,#26648),.UNSPECIFIED.,.F.,.F.)
B_SPLINE_CURVE_WITH_KNOTS((3,3),(0.136653338911782,0.195398016960283),
 .UNSPECIFIED.)
CURVE()
GEOMETRIC_REPRESENTATION_ITEM()
RATIONAL_B_SPLINE_CURVE((1.00492385476098,1.00359200155151,1.00020515445013))
REPRESENTATION_ITEM('')
);
#4109=LINE('',#26214,#5348);
#4110=LINE('',#26218,#5349);
#4111=LINE('',#26230,#5350);
#4112=LINE('',#26232,#5351);
#4113=LINE('',#26233,#5352);
#4114=LINE('',#26245,#5353);
#4115=LINE('',#26249,#5354);
#4116=LINE('',#26258,#5355);
#4117=LINE('',#26262,#5356);
#4118=LINE('',#26266,#5357);
#4119=LINE('',#26270,#5358);
#4120=LINE('',#26274,#5359);
#4121=LINE('',#26278,#5360);
#4122=LINE('',#26282,#5361);
#4123=LINE('',#26286,#5362);
#4124=LINE('',#26290,#5363);
#4125=LINE('',#26294,#5364);
#4126=LINE('',#26298,#5365);
#4127=LINE('',#26302,#5366);
#4128=LINE('',#26306,#5367);
#4129=LINE('',#26310,#5368);
#4130=LINE('',#26315,#5369);
#4131=LINE('',#26319,#5370);
#4132=LINE('',#26323,#5371);
#4133=LINE('',#26327,#5372);
#4134=LINE('',#26331,#5373);
#4135=LINE('',#26335,#5374);
#4136=LINE('',#26339,#5375);
#4137=LINE('',#26343,#5376);
#4138=LINE('',#26347,#5377);
#4139=LINE('',#26351,#5378);
#4140=LINE('',#26355,#5379);
#4141=LINE('',#26359,#5380);
#4142=LINE('',#26363,#5381);
#4143=LINE('',#26367,#5382);
#4144=LINE('',#26371,#5383);
#4145=LINE('',#26374,#5384);
#4146=LINE('',#26377,#5385);
#4147=LINE('',#26657,#5386);
#4148=LINE('',#26658,#5387);
#4149=LINE('',#26661,#5388);
#4150=LINE('',#26662,#5389);
#4151=LINE('',#26665,#5390);
#4152=LINE('',#26666,#5391);
#4153=LINE('',#26669,#5392);
#4154=LINE('',#26670,#5393);
#4155=LINE('',#26673,#5394);
#4156=LINE('',#26674,#5395);
#4157=LINE('',#26677,#5396);
#4158=LINE('',#26678,#5397);
#4159=LINE('',#26681,#5398);
#4160=LINE('',#26682,#5399);
#4161=LINE('',#26685,#5400);
#4162=LINE('',#26686,#5401);
#4163=LINE('',#26689,#5402);
#4164=LINE('',#26690,#5403);
#4165=LINE('',#26693,#5404);
#4166=LINE('',#26694,#5405);
#4167=LINE('',#26697,#5406);
#4168=LINE('',#26698,#5407);
#4169=LINE('',#26701,#5408);
#4170=LINE('',#26702,#5409);
#4171=LINE('',#26705,#5410);
#4172=LINE('',#26706,#5411);
#4173=LINE('',#26709,#5412);
#4174=LINE('',#26710,#5413);
#4175=LINE('',#26713,#5414);
#4176=LINE('',#26714,#5415);
#4177=LINE('',#26717,#5416);
#4178=LINE('',#26718,#5417);
#4179=LINE('',#26721,#5418);
#4180=LINE('',#26722,#5419);
#4181=LINE('',#26725,#5420);
#4182=LINE('',#26726,#5421);
#4183=LINE('',#26729,#5422);
#4184=LINE('',#26730,#5423);
#4185=LINE('',#26733,#5424);
#4186=LINE('',#26734,#5425);
#4187=LINE('',#26737,#5426);
#4188=LINE('',#26738,#5427);
#4189=LINE('',#26741,#5428);
#4190=LINE('',#26742,#5429);
#4191=LINE('',#26745,#5430);
#4192=LINE('',#26746,#5431);
#4193=LINE('',#26749,#5432);
#4194=LINE('',#26750,#5433);
#4195=LINE('',#26753,#5434);
#4196=LINE('',#26754,#5435);
#4197=LINE('',#26757,#5436);
#4198=LINE('',#26758,#5437);
#4199=LINE('',#26761,#5438);
#4200=LINE('',#26762,#5439);
#4201=LINE('',#26765,#5440);
#4202=LINE('',#26766,#5441);
#4203=LINE('',#26769,#5442);
#4204=LINE('',#26770,#5443);
#4205=LINE('',#26853,#5444);
#4206=LINE('',#26854,#5445);
#4207=LINE('',#26857,#5446);
#4208=LINE('',#26858,#5447);
#4209=LINE('',#26863,#5448);
#4210=LINE('',#26868,#5449);
#4211=LINE('',#26870,#5450);
#4212=LINE('',#26872,#5451);
#4213=LINE('',#26874,#5452);
#4214=LINE('',#26876,#5453);
#4215=LINE('',#26877,#5454);
#4216=LINE('',#26881,#5455);
#4217=LINE('',#26883,#5456);
#4218=LINE('',#26885,#5457);
#4219=LINE('',#26886,#5458);
#4220=LINE('',#26889,#5459);
#4221=LINE('',#26891,#5460);
#4222=LINE('',#26892,#5461);
#4223=LINE('',#26896,#5462);
#4224=LINE('',#26898,#5463);
#4225=LINE('',#26900,#5464);
#4226=LINE('',#26901,#5465);
#4227=LINE('',#26904,#5466);
#4228=LINE('',#26906,#5467);
#4229=LINE('',#26907,#5468);
#4230=LINE('',#26909,#5469);
#4231=LINE('',#26910,#5470);
#4232=LINE('',#26912,#5471);
#4233=LINE('',#26913,#5472);
#4234=LINE('',#26915,#5473);
#4235=LINE('',#26916,#5474);
#4236=LINE('',#26918,#5475);
#4237=LINE('',#26920,#5476);
#4238=LINE('',#26925,#5477);
#4239=LINE('',#26927,#5478);
#4240=LINE('',#26976,#5479);
#5348=VECTOR('',#18583,2.31);
#5349=VECTOR('',#18588,2.15);
#5350=VECTOR('',#18597,10.);
#5351=VECTOR('',#18598,10.);
#5352=VECTOR('',#18599,10.);
#5353=VECTOR('',#18606,10.);
#5354=VECTOR('',#18609,10.);
#5355=VECTOR('',#18612,10.);
#5356=VECTOR('',#18615,10.);
#5357=VECTOR('',#18618,10.);
#5358=VECTOR('',#18621,10.);
#5359=VECTOR('',#18624,10.);
#5360=VECTOR('',#18627,10.);
#5361=VECTOR('',#18630,10.);
#5362=VECTOR('',#18633,10.);
#5363=VECTOR('',#18636,10.);
#5364=VECTOR('',#18639,10.);
#5365=VECTOR('',#18642,10.);
#5366=VECTOR('',#18645,10.);
#5367=VECTOR('',#18648,10.);
#5368=VECTOR('',#18651,6.5);
#5369=VECTOR('',#18656,10.);
#5370=VECTOR('',#18659,10.);
#5371=VECTOR('',#18662,10.);
#5372=VECTOR('',#18665,10.);
#5373=VECTOR('',#18668,10.);
#5374=VECTOR('',#18671,10.);
#5375=VECTOR('',#18674,10.);
#5376=VECTOR('',#18677,10.);
#5377=VECTOR('',#18680,10.);
#5378=VECTOR('',#18683,10.);
#5379=VECTOR('',#18686,10.);
#5380=VECTOR('',#18689,10.);
#5381=VECTOR('',#18692,10.);
#5382=VECTOR('',#18695,10.);
#5383=VECTOR('',#18698,10.);
#5384=VECTOR('',#18701,10.);
#5385=VECTOR('',#18704,6.2);
#5386=VECTOR('',#18707,10.);
#5387=VECTOR('',#18708,10.);
#5388=VECTOR('',#18711,10.);
#5389=VECTOR('',#18712,10.);
#5390=VECTOR('',#18715,10.);
#5391=VECTOR('',#18716,10.);
#5392=VECTOR('',#18719,10.);
#5393=VECTOR('',#18720,10.);
#5394=VECTOR('',#18723,10.);
#5395=VECTOR('',#18724,10.);
#5396=VECTOR('',#18727,10.);
#5397=VECTOR('',#18728,10.);
#5398=VECTOR('',#18731,10.);
#5399=VECTOR('',#18732,10.);
#5400=VECTOR('',#18735,10.);
#5401=VECTOR('',#18736,10.);
#5402=VECTOR('',#18739,10.);
#5403=VECTOR('',#18740,10.);
#5404=VECTOR('',#18743,10.);
#5405=VECTOR('',#18744,10.);
#5406=VECTOR('',#18747,10.);
#5407=VECTOR('',#18748,10.);
#5408=VECTOR('',#18751,10.);
#5409=VECTOR('',#18752,10.);
#5410=VECTOR('',#18755,10.);
#5411=VECTOR('',#18756,10.);
#5412=VECTOR('',#18759,10.);
#5413=VECTOR('',#18760,10.);
#5414=VECTOR('',#18763,10.);
#5415=VECTOR('',#18764,10.);
#5416=VECTOR('',#18767,10.);
#5417=VECTOR('',#18768,10.);
#5418=VECTOR('',#18771,10.);
#5419=VECTOR('',#18772,10.);
#5420=VECTOR('',#18775,10.);
#5421=VECTOR('',#18776,10.);
#5422=VECTOR('',#18779,10.);
#5423=VECTOR('',#18780,10.);
#5424=VECTOR('',#18783,10.);
#5425=VECTOR('',#18784,10.);
#5426=VECTOR('',#18787,10.);
#5427=VECTOR('',#18788,10.);
#5428=VECTOR('',#18791,10.);
#5429=VECTOR('',#18792,10.);
#5430=VECTOR('',#18795,10.);
#5431=VECTOR('',#18796,10.);
#5432=VECTOR('',#18799,10.);
#5433=VECTOR('',#18800,10.);
#5434=VECTOR('',#18803,10.);
#5435=VECTOR('',#18804,10.);
#5436=VECTOR('',#18807,10.);
#5437=VECTOR('',#18808,10.);
#5438=VECTOR('',#18811,10.);
#5439=VECTOR('',#18812,10.);
#5440=VECTOR('',#18815,10.);
#5441=VECTOR('',#18816,10.);
#5442=VECTOR('',#18819,10.);
#5443=VECTOR('',#18820,10.);
#5444=VECTOR('',#18823,10.);
#5445=VECTOR('',#18824,10.);
#5446=VECTOR('',#18827,10.);
#5447=VECTOR('',#18828,10.);
#5448=VECTOR('',#18835,2.31);
#5449=VECTOR('',#18840,10.);
#5450=VECTOR('',#18841,10.);
#5451=VECTOR('',#18842,10.);
#5452=VECTOR('',#18843,10.);
#5453=VECTOR('',#18844,10.);
#5454=VECTOR('',#18845,10.);
#5455=VECTOR('',#18848,10.);
#5456=VECTOR('',#18849,10.);
#5457=VECTOR('',#18850,10.);
#5458=VECTOR('',#18851,10.);
#5459=VECTOR('',#18854,10.);
#5460=VECTOR('',#18855,10.);
#5461=VECTOR('',#18856,10.);
#5462=VECTOR('',#18859,10.);
#5463=VECTOR('',#18860,10.);
#5464=VECTOR('',#18861,10.);
#5465=VECTOR('',#18862,10.);
#5466=VECTOR('',#18865,10.);
#5467=VECTOR('',#18866,10.);
#5468=VECTOR('',#18867,10.);
#5469=VECTOR('',#18870,10.);
#5470=VECTOR('',#18871,10.);
#5471=VECTOR('',#18874,10.);
#5472=VECTOR('',#18875,10.);
#5473=VECTOR('',#18878,10.);
#5474=VECTOR('',#18879,10.);
#5475=VECTOR('',#18882,10.);
#5476=VECTOR('',#18885,10.);
#5477=VECTOR('',#18892,10.);
#5478=VECTOR('',#18895,10.);
#5479=VECTOR('',#18992,6.25);
#6480=VERTEX_POINT('',#26209);
#6481=VERTEX_POINT('',#26210);
#6482=VERTEX_POINT('',#26213);
#6483=VERTEX_POINT('',#26217);
#6484=VERTEX_POINT('',#26221);
#6485=VERTEX_POINT('',#26224);
#6486=VERTEX_POINT('',#26225);
#6487=VERTEX_POINT('',#26229);
#6488=VERTEX_POINT('',#26231);
#6489=VERTEX_POINT('',#26235);
#6490=VERTEX_POINT('',#26237);
#6491=VERTEX_POINT('',#26239);
#6492=VERTEX_POINT('',#26244);
#6493=VERTEX_POINT('',#26246);
#6494=VERTEX_POINT('',#26248);
#6495=VERTEX_POINT('',#26250);
#6496=VERTEX_POINT('',#26255);
#6497=VERTEX_POINT('',#26257);
#6498=VERTEX_POINT('',#26259);
#6499=VERTEX_POINT('',#26261);
#6500=VERTEX_POINT('',#26263);
#6501=VERTEX_POINT('',#26265);
#6502=VERTEX_POINT('',#26267);
#6503=VERTEX_POINT('',#26269);
#6504=VERTEX_POINT('',#26271);
#6505=VERTEX_POINT('',#26273);
#6506=VERTEX_POINT('',#26275);
#6507=VERTEX_POINT('',#26277);
#6508=VERTEX_POINT('',#26279);
#6509=VERTEX_POINT('',#26281);
#6510=VERTEX_POINT('',#26283);
#6511=VERTEX_POINT('',#26285);
#6512=VERTEX_POINT('',#26287);
#6513=VERTEX_POINT('',#26289);
#6514=VERTEX_POINT('',#26291);
#6515=VERTEX_POINT('',#26293);
#6516=VERTEX_POINT('',#26295);
#6517=VERTEX_POINT('',#26297);
#6518=VERTEX_POINT('',#26299);
#6519=VERTEX_POINT('',#26301);
#6520=VERTEX_POINT('',#26303);
#6521=VERTEX_POINT('',#26305);
#6522=VERTEX_POINT('',#26307);
#6523=VERTEX_POINT('',#26309);
#6524=VERTEX_POINT('',#26312);
#6525=VERTEX_POINT('',#26314);
#6526=VERTEX_POINT('',#26316);
#6527=VERTEX_POINT('',#26318);
#6528=VERTEX_POINT('',#26320);
#6529=VERTEX_POINT('',#26322);
#6530=VERTEX_POINT('',#26324);
#6531=VERTEX_POINT('',#26326);
#6532=VERTEX_POINT('',#26328);
#6533=VERTEX_POINT('',#26330);
#6534=VERTEX_POINT('',#26332);
#6535=VERTEX_POINT('',#26334);
#6536=VERTEX_POINT('',#26336);
#6537=VERTEX_POINT('',#26338);
#6538=VERTEX_POINT('',#26340);
#6539=VERTEX_POINT('',#26342);
#6540=VERTEX_POINT('',#26344);
#6541=VERTEX_POINT('',#26346);
#6542=VERTEX_POINT('',#26348);
#6543=VERTEX_POINT('',#26350);
#6544=VERTEX_POINT('',#26352);
#6545=VERTEX_POINT('',#26354);
#6546=VERTEX_POINT('',#26356);
#6547=VERTEX_POINT('',#26358);
#6548=VERTEX_POINT('',#26360);
#6549=VERTEX_POINT('',#26362);
#6550=VERTEX_POINT('',#26364);
#6551=VERTEX_POINT('',#26366);
#6552=VERTEX_POINT('',#26368);
#6553=VERTEX_POINT('',#26370);
#6554=VERTEX_POINT('',#26372);
#6555=VERTEX_POINT('',#26376);
#6556=VERTEX_POINT('',#26378);
#6557=VERTEX_POINT('',#26388);
#6558=VERTEX_POINT('',#26392);
#6559=VERTEX_POINT('',#26406);
#6560=VERTEX_POINT('',#26410);
#6561=VERTEX_POINT('',#26424);
#6562=VERTEX_POINT('',#26428);
#6563=VERTEX_POINT('',#26442);
#6564=VERTEX_POINT('',#26446);
#6565=VERTEX_POINT('',#26460);
#6566=VERTEX_POINT('',#26464);
#6567=VERTEX_POINT('',#26478);
#6568=VERTEX_POINT('',#26482);
#6569=VERTEX_POINT('',#26505);
#6570=VERTEX_POINT('',#26519);
#6571=VERTEX_POINT('',#26523);
#6572=VERTEX_POINT('',#26537);
#6573=VERTEX_POINT('',#26541);
#6574=VERTEX_POINT('',#26555);
#6575=VERTEX_POINT('',#26559);
#6576=VERTEX_POINT('',#26573);
#6577=VERTEX_POINT('',#26577);
#6578=VERTEX_POINT('',#26591);
#6579=VERTEX_POINT('',#26595);
#6580=VERTEX_POINT('',#26609);
#6581=VERTEX_POINT('',#26613);
#6582=VERTEX_POINT('',#26627);
#6583=VERTEX_POINT('',#26631);
#6584=VERTEX_POINT('',#26645);
#6585=VERTEX_POINT('',#26656);
#6586=VERTEX_POINT('',#26660);
#6587=VERTEX_POINT('',#26664);
#6588=VERTEX_POINT('',#26668);
#6589=VERTEX_POINT('',#26672);
#6590=VERTEX_POINT('',#26676);
#6591=VERTEX_POINT('',#26680);
#6592=VERTEX_POINT('',#26684);
#6593=VERTEX_POINT('',#26688);
#6594=VERTEX_POINT('',#26692);
#6595=VERTEX_POINT('',#26696);
#6596=VERTEX_POINT('',#26700);
#6597=VERTEX_POINT('',#26704);
#6598=VERTEX_POINT('',#26708);
#6599=VERTEX_POINT('',#26712);
#6600=VERTEX_POINT('',#26716);
#6601=VERTEX_POINT('',#26720);
#6602=VERTEX_POINT('',#26724);
#6603=VERTEX_POINT('',#26728);
#6604=VERTEX_POINT('',#26732);
#6605=VERTEX_POINT('',#26736);
#6606=VERTEX_POINT('',#26740);
#6607=VERTEX_POINT('',#26744);
#6608=VERTEX_POINT('',#26748);
#6609=VERTEX_POINT('',#26752);
#6610=VERTEX_POINT('',#26756);
#6611=VERTEX_POINT('',#26760);
#6612=VERTEX_POINT('',#26764);
#6613=VERTEX_POINT('',#26768);
#6614=VERTEX_POINT('',#26807);
#6615=VERTEX_POINT('',#26808);
#6616=VERTEX_POINT('',#26852);
#6617=VERTEX_POINT('',#26856);
#6618=VERTEX_POINT('',#26862);
#6619=VERTEX_POINT('',#26866);
#6620=VERTEX_POINT('',#26867);
#6621=VERTEX_POINT('',#26869);
#6622=VERTEX_POINT('',#26871);
#6623=VERTEX_POINT('',#26873);
#6624=VERTEX_POINT('',#26875);
#6625=VERTEX_POINT('',#26879);
#6626=VERTEX_POINT('',#26880);
#6627=VERTEX_POINT('',#26882);
#6628=VERTEX_POINT('',#26884);
#6629=VERTEX_POINT('',#26888);
#6630=VERTEX_POINT('',#26890);
#6631=VERTEX_POINT('',#26894);
#6632=VERTEX_POINT('',#26895);
#6633=VERTEX_POINT('',#26897);
#6634=VERTEX_POINT('',#26899);
#6635=VERTEX_POINT('',#26903);
#6636=VERTEX_POINT('',#26905);
#6637=VERTEX_POINT('',#26922);
#8343=EDGE_CURVE('',#6480,#6481,#1182,.T.);
#8344=EDGE_CURVE('',#6481,#6480,#1183,.T.);
#8345=EDGE_CURVE('',#6480,#6482,#4109,.T.);
#8346=EDGE_CURVE('',#6482,#6482,#1184,.T.);
#8347=EDGE_CURVE('',#6481,#6483,#4110,.T.);
#8348=EDGE_CURVE('',#6483,#6483,#1185,.T.);
#8349=EDGE_CURVE('',#6484,#6484,#1186,.T.);
#8350=EDGE_CURVE('',#6485,#6486,#3138,.T.);
#8351=EDGE_CURVE('',#6486,#6487,#4111,.T.);
#8352=EDGE_CURVE('',#6487,#6488,#4112,.F.);
#8353=EDGE_CURVE('',#6488,#6485,#4113,.T.);
#8354=EDGE_CURVE('',#6489,#6487,#1187,.T.);
#8355=EDGE_CURVE('',#6490,#6486,#1188,.T.);
#8356=EDGE_CURVE('',#6491,#6490,#259,.T.);
#8357=EDGE_CURVE('',#6492,#6491,#4114,.T.);
#8358=EDGE_CURVE('',#6492,#6493,#1189,.T.);
#8359=EDGE_CURVE('',#6494,#6493,#4115,.T.);
#8360=EDGE_CURVE('',#6495,#6494,#260,.T.);
#8361=EDGE_CURVE('',#6496,#6495,#1190,.T.);
#8362=EDGE_CURVE('',#6497,#6496,#4116,.T.);
#8363=EDGE_CURVE('',#6497,#6498,#1191,.T.);
#8364=EDGE_CURVE('',#6499,#6498,#4117,.T.);
#8365=EDGE_CURVE('',#6500,#6499,#1192,.T.);
#8366=EDGE_CURVE('',#6501,#6500,#4118,.T.);
#8367=EDGE_CURVE('',#6501,#6502,#1193,.T.);
#8368=EDGE_CURVE('',#6503,#6502,#4119,.T.);
#8369=EDGE_CURVE('',#6504,#6503,#1194,.T.);
#8370=EDGE_CURVE('',#6505,#6504,#4120,.T.);
#8371=EDGE_CURVE('',#6505,#6506,#1195,.T.);
#8372=EDGE_CURVE('',#6507,#6506,#4121,.T.);
#8373=EDGE_CURVE('',#6508,#6507,#1196,.T.);
#8374=EDGE_CURVE('',#6509,#6508,#4122,.T.);
#8375=EDGE_CURVE('',#6509,#6510,#1197,.T.);
#8376=EDGE_CURVE('',#6511,#6510,#4123,.T.);
#8377=EDGE_CURVE('',#6512,#6511,#1198,.T.);
#8378=EDGE_CURVE('',#6513,#6512,#4124,.T.);
#8379=EDGE_CURVE('',#6513,#6514,#1199,.T.);
#8380=EDGE_CURVE('',#6515,#6514,#4125,.T.);
#8381=EDGE_CURVE('',#6516,#6515,#1200,.T.);
#8382=EDGE_CURVE('',#6517,#6516,#4126,.T.);
#8383=EDGE_CURVE('',#6517,#6518,#1201,.T.);
#8384=EDGE_CURVE('',#6519,#6518,#4127,.T.);
#8385=EDGE_CURVE('',#6520,#6519,#1202,.T.);
#8386=EDGE_CURVE('',#6521,#6520,#4128,.T.);
#8387=EDGE_CURVE('',#6521,#6522,#1203,.T.);
#8388=EDGE_CURVE('',#6522,#6523,#4129,.T.);
#8389=EDGE_CURVE('',#6523,#6523,#1204,.T.);
#8390=EDGE_CURVE('',#6522,#6524,#1205,.T.);
#8391=EDGE_CURVE('',#6525,#6524,#4130,.T.);
#8392=EDGE_CURVE('',#6526,#6525,#1206,.T.);
#8393=EDGE_CURVE('',#6527,#6526,#4131,.T.);
#8394=EDGE_CURVE('',#6527,#6528,#1207,.T.);
#8395=EDGE_CURVE('',#6529,#6528,#4132,.T.);
#8396=EDGE_CURVE('',#6530,#6529,#1208,.T.);
#8397=EDGE_CURVE('',#6531,#6530,#4133,.T.);
#8398=EDGE_CURVE('',#6531,#6532,#1209,.T.);
#8399=EDGE_CURVE('',#6533,#6532,#4134,.T.);
#8400=EDGE_CURVE('',#6534,#6533,#1210,.T.);
#8401=EDGE_CURVE('',#6535,#6534,#4135,.T.);
#8402=EDGE_CURVE('',#6535,#6536,#1211,.T.);
#8403=EDGE_CURVE('',#6537,#6536,#4136,.T.);
#8404=EDGE_CURVE('',#6538,#6537,#1212,.T.);
#8405=EDGE_CURVE('',#6539,#6538,#4137,.T.);
#8406=EDGE_CURVE('',#6539,#6540,#1213,.T.);
#8407=EDGE_CURVE('',#6541,#6540,#4138,.T.);
#8408=EDGE_CURVE('',#6542,#6541,#1214,.T.);
#8409=EDGE_CURVE('',#6543,#6542,#4139,.T.);
#8410=EDGE_CURVE('',#6543,#6544,#1215,.T.);
#8411=EDGE_CURVE('',#6545,#6544,#4140,.T.);
#8412=EDGE_CURVE('',#6546,#6545,#1216,.T.);
#8413=EDGE_CURVE('',#6547,#6546,#4141,.T.);
#8414=EDGE_CURVE('',#6547,#6548,#1217,.T.);
#8415=EDGE_CURVE('',#6549,#6548,#4142,.T.);
#8416=EDGE_CURVE('',#6550,#6549,#1218,.T.);
#8417=EDGE_CURVE('',#6551,#6550,#4143,.T.);
#8418=EDGE_CURVE('',#6551,#6552,#1219,.T.);
#8419=EDGE_CURVE('',#6553,#6552,#4144,.T.);
#8420=EDGE_CURVE('',#6554,#6553,#1220,.T.);
#8421=EDGE_CURVE('',#6489,#6554,#4145,.T.);
#8422=EDGE_CURVE('',#6484,#6555,#4146,.T.);
#8423=EDGE_CURVE('',#6555,#6556,#261,.T.);
#8424=EDGE_CURVE('',#6520,#6556,#3139,.T.);
#8425=EDGE_CURVE('',#6557,#6519,#3140,.T.);
#8426=EDGE_CURVE('',#6557,#6558,#262,.T.);
#8427=EDGE_CURVE('',#6516,#6558,#3141,.T.);
#8428=EDGE_CURVE('',#6559,#6515,#3142,.T.);
#8429=EDGE_CURVE('',#6559,#6560,#263,.T.);
#8430=EDGE_CURVE('',#6512,#6560,#3143,.T.);
#8431=EDGE_CURVE('',#6561,#6511,#3144,.T.);
#8432=EDGE_CURVE('',#6561,#6562,#264,.T.);
#8433=EDGE_CURVE('',#6508,#6562,#3145,.T.);
#8434=EDGE_CURVE('',#6563,#6507,#3146,.T.);
#8435=EDGE_CURVE('',#6563,#6564,#265,.T.);
#8436=EDGE_CURVE('',#6504,#6564,#3147,.T.);
#8437=EDGE_CURVE('',#6565,#6503,#3148,.T.);
#8438=EDGE_CURVE('',#6565,#6566,#266,.T.);
#8439=EDGE_CURVE('',#6500,#6566,#3149,.T.);
#8440=EDGE_CURVE('',#6567,#6499,#3150,.T.);
#8441=EDGE_CURVE('',#6567,#6568,#267,.T.);
#8442=EDGE_CURVE('',#6496,#6568,#3151,.T.);
#8443=EDGE_CURVE('',#6490,#6495,#268,.T.);
#8444=EDGE_CURVE('',#6485,#6569,#269,.T.);
#8445=EDGE_CURVE('',#6554,#6569,#3152,.T.);
#8446=EDGE_CURVE('',#6570,#6553,#3153,.T.);
#8447=EDGE_CURVE('',#6570,#6571,#270,.T.);
#8448=EDGE_CURVE('',#6550,#6571,#3154,.T.);
#8449=EDGE_CURVE('',#6572,#6549,#3155,.T.);
#8450=EDGE_CURVE('',#6572,#6573,#271,.T.);
#8451=EDGE_CURVE('',#6546,#6573,#3156,.T.);
#8452=EDGE_CURVE('',#6574,#6545,#3157,.T.);
#8453=EDGE_CURVE('',#6574,#6575,#272,.T.);
#8454=EDGE_CURVE('',#6542,#6575,#3158,.T.);
#8455=EDGE_CURVE('',#6576,#6541,#3159,.T.);
#8456=EDGE_CURVE('',#6576,#6577,#273,.T.);
#8457=EDGE_CURVE('',#6538,#6577,#3160,.T.);
#8458=EDGE_CURVE('',#6578,#6537,#3161,.T.);
#8459=EDGE_CURVE('',#6578,#6579,#274,.T.);
#8460=EDGE_CURVE('',#6534,#6579,#3162,.T.);
#8461=EDGE_CURVE('',#6580,#6533,#3163,.T.);
#8462=EDGE_CURVE('',#6580,#6581,#275,.T.);
#8463=EDGE_CURVE('',#6530,#6581,#3164,.T.);
#8464=EDGE_CURVE('',#6582,#6529,#3165,.T.);
#8465=EDGE_CURVE('',#6582,#6583,#276,.T.);
#8466=EDGE_CURVE('',#6526,#6583,#3166,.T.);
#8467=EDGE_CURVE('',#6584,#6525,#3167,.T.);
#8468=EDGE_CURVE('',#6584,#6555,#277,.T.);
#8469=EDGE_CURVE('',#6569,#6585,#4147,.T.);
#8470=EDGE_CURVE('',#6585,#6489,#4148,.F.);
#8471=EDGE_CURVE('',#6552,#6586,#4149,.F.);
#8472=EDGE_CURVE('',#6586,#6570,#4150,.T.);
#8473=EDGE_CURVE('',#6571,#6587,#4151,.T.);
#8474=EDGE_CURVE('',#6587,#6551,#4152,.F.);
#8475=EDGE_CURVE('',#6548,#6588,#4153,.F.);
#8476=EDGE_CURVE('',#6588,#6572,#4154,.T.);
#8477=EDGE_CURVE('',#6573,#6589,#4155,.T.);
#8478=EDGE_CURVE('',#6589,#6547,#4156,.F.);
#8479=EDGE_CURVE('',#6544,#6590,#4157,.F.);
#8480=EDGE_CURVE('',#6590,#6574,#4158,.T.);
#8481=EDGE_CURVE('',#6575,#6591,#4159,.T.);
#8482=EDGE_CURVE('',#6591,#6543,#4160,.F.);
#8483=EDGE_CURVE('',#6540,#6592,#4161,.F.);
#8484=EDGE_CURVE('',#6592,#6576,#4162,.T.);
#8485=EDGE_CURVE('',#6577,#6593,#4163,.T.);
#8486=EDGE_CURVE('',#6593,#6539,#4164,.F.);
#8487=EDGE_CURVE('',#6536,#6594,#4165,.F.);
#8488=EDGE_CURVE('',#6594,#6578,#4166,.T.);
#8489=EDGE_CURVE('',#6579,#6595,#4167,.T.);
#8490=EDGE_CURVE('',#6595,#6535,#4168,.F.);
#8491=EDGE_CURVE('',#6532,#6596,#4169,.F.);
#8492=EDGE_CURVE('',#6596,#6580,#4170,.T.);
#8493=EDGE_CURVE('',#6581,#6597,#4171,.T.);
#8494=EDGE_CURVE('',#6597,#6531,#4172,.F.);
#8495=EDGE_CURVE('',#6528,#6598,#4173,.F.);
#8496=EDGE_CURVE('',#6598,#6582,#4174,.T.);
#8497=EDGE_CURVE('',#6583,#6599,#4175,.T.);
#8498=EDGE_CURVE('',#6599,#6527,#4176,.F.);
#8499=EDGE_CURVE('',#6524,#6600,#4177,.F.);
#8500=EDGE_CURVE('',#6600,#6584,#4178,.T.);
#8501=EDGE_CURVE('',#6556,#6601,#4179,.T.);
#8502=EDGE_CURVE('',#6601,#6521,#4180,.F.);
#8503=EDGE_CURVE('',#6518,#6602,#4181,.F.);
#8504=EDGE_CURVE('',#6602,#6557,#4182,.T.);
#8505=EDGE_CURVE('',#6558,#6603,#4183,.T.);
#8506=EDGE_CURVE('',#6603,#6517,#4184,.F.);
#8507=EDGE_CURVE('',#6514,#6604,#4185,.F.);
#8508=EDGE_CURVE('',#6604,#6559,#4186,.T.);
#8509=EDGE_CURVE('',#6560,#6605,#4187,.T.);
#8510=EDGE_CURVE('',#6605,#6513,#4188,.F.);
#8511=EDGE_CURVE('',#6510,#6606,#4189,.F.);
#8512=EDGE_CURVE('',#6606,#6561,#4190,.T.);
#8513=EDGE_CURVE('',#6562,#6607,#4191,.T.);
#8514=EDGE_CURVE('',#6607,#6509,#4192,.F.);
#8515=EDGE_CURVE('',#6506,#6608,#4193,.F.);
#8516=EDGE_CURVE('',#6608,#6563,#4194,.T.);
#8517=EDGE_CURVE('',#6564,#6609,#4195,.T.);
#8518=EDGE_CURVE('',#6609,#6505,#4196,.F.);
#8519=EDGE_CURVE('',#6502,#6610,#4197,.F.);
#8520=EDGE_CURVE('',#6610,#6565,#4198,.T.);
#8521=EDGE_CURVE('',#6566,#6611,#4199,.T.);
#8522=EDGE_CURVE('',#6611,#6501,#4200,.F.);
#8523=EDGE_CURVE('',#6498,#6612,#4201,.F.);
#8524=EDGE_CURVE('',#6612,#6567,#4202,.T.);
#8525=EDGE_CURVE('',#6568,#6613,#4203,.T.);
#8526=EDGE_CURVE('',#6613,#6497,#4204,.F.);
#8527=EDGE_CURVE('',#6614,#6615,#278,.T.);
#8528=EDGE_CURVE('',#6615,#6491,#279,.T.);
#8529=EDGE_CURVE('',#6494,#6614,#280,.T.);
#8530=EDGE_CURVE('',#6615,#6616,#4205,.T.);
#8531=EDGE_CURVE('',#6616,#6492,#4206,.F.);
#8532=EDGE_CURVE('',#6493,#6617,#4207,.F.);
#8533=EDGE_CURVE('',#6617,#6614,#4208,.T.);
#8534=EDGE_CURVE('',#6616,#6617,#1221,.T.);
#8535=EDGE_CURVE('',#6483,#6618,#4209,.T.);
#8536=EDGE_CURVE('',#6618,#6618,#1222,.T.);
#8537=EDGE_CURVE('',#6619,#6620,#4210,.T.);
#8538=EDGE_CURVE('',#6621,#6619,#4211,.T.);
#8539=EDGE_CURVE('',#6622,#6621,#4212,.T.);
#8540=EDGE_CURVE('',#6623,#6622,#4213,.T.);
#8541=EDGE_CURVE('',#6624,#6623,#4214,.T.);
#8542=EDGE_CURVE('',#6620,#6624,#4215,.T.);
#8543=EDGE_CURVE('',#6625,#6626,#4216,.T.);
#8544=EDGE_CURVE('',#6626,#6627,#4217,.T.);
#8545=EDGE_CURVE('',#6627,#6628,#4218,.T.);
#8546=EDGE_CURVE('',#6625,#6628,#4219,.T.);
#8547=EDGE_CURVE('',#6626,#6629,#4220,.T.);
#8548=EDGE_CURVE('',#6629,#6630,#4221,.T.);
#8549=EDGE_CURVE('',#6630,#6627,#4222,.T.);
#8550=EDGE_CURVE('',#6631,#6632,#4223,.T.);
#8551=EDGE_CURVE('',#6632,#6633,#4224,.T.);
#8552=EDGE_CURVE('',#6633,#6634,#4225,.T.);
#8553=EDGE_CURVE('',#6634,#6631,#4226,.T.);
#8554=EDGE_CURVE('',#6635,#6633,#4227,.T.);
#8555=EDGE_CURVE('',#6632,#6636,#4228,.T.);
#8556=EDGE_CURVE('',#6636,#6635,#4229,.T.);
#8557=EDGE_CURVE('',#6629,#6631,#4230,.T.);
#8558=EDGE_CURVE('',#6634,#6630,#4231,.T.);
#8559=EDGE_CURVE('',#6628,#6635,#4232,.T.);
#8560=EDGE_CURVE('',#6636,#6625,#4233,.T.);
#8561=EDGE_CURVE('',#6630,#6620,#4234,.T.);
#8562=EDGE_CURVE('',#6627,#6624,#4235,.T.);
#8563=EDGE_CURVE('',#6634,#6619,#4236,.T.);
#8564=EDGE_CURVE('',#6633,#6621,#4237,.T.);
#8565=EDGE_CURVE('',#6637,#6637,#1223,.T.);
#8566=EDGE_CURVE('',#6635,#6622,#4238,.T.);
#8567=EDGE_CURVE('',#6628,#6623,#4239,.T.);
#8568=EDGE_CURVE('',#6613,#6612,#1224,.T.);
#8569=EDGE_CURVE('',#6611,#6610,#1225,.T.);
#8570=EDGE_CURVE('',#6609,#6608,#1226,.T.);
#8571=EDGE_CURVE('',#6607,#6606,#1227,.T.);
#8572=EDGE_CURVE('',#6605,#6604,#1228,.T.);
#8573=EDGE_CURVE('',#6603,#6602,#1229,.T.);
#8574=EDGE_CURVE('',#6601,#6600,#1230,.T.);
#8575=EDGE_CURVE('',#6599,#6598,#1231,.T.);
#8576=EDGE_CURVE('',#6597,#6596,#1232,.T.);
#8577=EDGE_CURVE('',#6595,#6594,#1233,.T.);
#8578=EDGE_CURVE('',#6593,#6592,#1234,.T.);
#8579=EDGE_CURVE('',#6591,#6590,#1235,.T.);
#8580=EDGE_CURVE('',#6589,#6588,#1236,.T.);
#8581=EDGE_CURVE('',#6587,#6586,#1237,.T.);
#8582=EDGE_CURVE('',#6585,#6488,#1238,.T.);
#8583=EDGE_CURVE('',#6523,#6637,#4240,.T.);
#11803=ORIENTED_EDGE('',*,*,#8343,.T.);
#11804=ORIENTED_EDGE('',*,*,#8344,.T.);
#11805=ORIENTED_EDGE('',*,*,#8345,.T.);
#11806=ORIENTED_EDGE('',*,*,#8346,.T.);
#11807=ORIENTED_EDGE('',*,*,#8345,.F.);
#11808=ORIENTED_EDGE('',*,*,#8343,.F.);
#11809=ORIENTED_EDGE('',*,*,#8344,.F.);
#11810=ORIENTED_EDGE('',*,*,#8347,.T.);
#11811=ORIENTED_EDGE('',*,*,#8348,.F.);
#11812=ORIENTED_EDGE('',*,*,#8347,.F.);
#11813=ORIENTED_EDGE('',*,*,#8349,.T.);
#11814=ORIENTED_EDGE('',*,*,#8346,.F.);
#11815=ORIENTED_EDGE('',*,*,#8350,.T.);
#11816=ORIENTED_EDGE('',*,*,#8351,.T.);
#11817=ORIENTED_EDGE('',*,*,#8352,.T.);
#11818=ORIENTED_EDGE('',*,*,#8353,.T.);
#11819=ORIENTED_EDGE('',*,*,#8354,.T.);
#11820=ORIENTED_EDGE('',*,*,#8351,.F.);
#11821=ORIENTED_EDGE('',*,*,#8355,.F.);
#11822=ORIENTED_EDGE('',*,*,#8356,.F.);
#11823=ORIENTED_EDGE('',*,*,#8357,.F.);
#11824=ORIENTED_EDGE('',*,*,#8358,.T.);
#11825=ORIENTED_EDGE('',*,*,#8359,.F.);
#11826=ORIENTED_EDGE('',*,*,#8360,.F.);
#11827=ORIENTED_EDGE('',*,*,#8361,.F.);
#11828=ORIENTED_EDGE('',*,*,#8362,.F.);
#11829=ORIENTED_EDGE('',*,*,#8363,.T.);
#11830=ORIENTED_EDGE('',*,*,#8364,.F.);
#11831=ORIENTED_EDGE('',*,*,#8365,.F.);
#11832=ORIENTED_EDGE('',*,*,#8366,.F.);
#11833=ORIENTED_EDGE('',*,*,#8367,.T.);
#11834=ORIENTED_EDGE('',*,*,#8368,.F.);
#11835=ORIENTED_EDGE('',*,*,#8369,.F.);
#11836=ORIENTED_EDGE('',*,*,#8370,.F.);
#11837=ORIENTED_EDGE('',*,*,#8371,.T.);
#11838=ORIENTED_EDGE('',*,*,#8372,.F.);
#11839=ORIENTED_EDGE('',*,*,#8373,.F.);
#11840=ORIENTED_EDGE('',*,*,#8374,.F.);
#11841=ORIENTED_EDGE('',*,*,#8375,.T.);
#11842=ORIENTED_EDGE('',*,*,#8376,.F.);
#11843=ORIENTED_EDGE('',*,*,#8377,.F.);
#11844=ORIENTED_EDGE('',*,*,#8378,.F.);
#11845=ORIENTED_EDGE('',*,*,#8379,.T.);
#11846=ORIENTED_EDGE('',*,*,#8380,.F.);
#11847=ORIENTED_EDGE('',*,*,#8381,.F.);
#11848=ORIENTED_EDGE('',*,*,#8382,.F.);
#11849=ORIENTED_EDGE('',*,*,#8383,.T.);
#11850=ORIENTED_EDGE('',*,*,#8384,.F.);
#11851=ORIENTED_EDGE('',*,*,#8385,.F.);
#11852=ORIENTED_EDGE('',*,*,#8386,.F.);
#11853=ORIENTED_EDGE('',*,*,#8387,.T.);
#11854=ORIENTED_EDGE('',*,*,#8388,.T.);
#11855=ORIENTED_EDGE('',*,*,#8389,.T.);
#11856=ORIENTED_EDGE('',*,*,#8388,.F.);
#11857=ORIENTED_EDGE('',*,*,#8390,.T.);
#11858=ORIENTED_EDGE('',*,*,#8391,.F.);
#11859=ORIENTED_EDGE('',*,*,#8392,.F.);
#11860=ORIENTED_EDGE('',*,*,#8393,.F.);
#11861=ORIENTED_EDGE('',*,*,#8394,.T.);
#11862=ORIENTED_EDGE('',*,*,#8395,.F.);
#11863=ORIENTED_EDGE('',*,*,#8396,.F.);
#11864=ORIENTED_EDGE('',*,*,#8397,.F.);
#11865=ORIENTED_EDGE('',*,*,#8398,.T.);
#11866=ORIENTED_EDGE('',*,*,#8399,.F.);
#11867=ORIENTED_EDGE('',*,*,#8400,.F.);
#11868=ORIENTED_EDGE('',*,*,#8401,.F.);
#11869=ORIENTED_EDGE('',*,*,#8402,.T.);
#11870=ORIENTED_EDGE('',*,*,#8403,.F.);
#11871=ORIENTED_EDGE('',*,*,#8404,.F.);
#11872=ORIENTED_EDGE('',*,*,#8405,.F.);
#11873=ORIENTED_EDGE('',*,*,#8406,.T.);
#11874=ORIENTED_EDGE('',*,*,#8407,.F.);
#11875=ORIENTED_EDGE('',*,*,#8408,.F.);
#11876=ORIENTED_EDGE('',*,*,#8409,.F.);
#11877=ORIENTED_EDGE('',*,*,#8410,.T.);
#11878=ORIENTED_EDGE('',*,*,#8411,.F.);
#11879=ORIENTED_EDGE('',*,*,#8412,.F.);
#11880=ORIENTED_EDGE('',*,*,#8413,.F.);
#11881=ORIENTED_EDGE('',*,*,#8414,.T.);
#11882=ORIENTED_EDGE('',*,*,#8415,.F.);
#11883=ORIENTED_EDGE('',*,*,#8416,.F.);
#11884=ORIENTED_EDGE('',*,*,#8417,.F.);
#11885=ORIENTED_EDGE('',*,*,#8418,.T.);
#11886=ORIENTED_EDGE('',*,*,#8419,.F.);
#11887=ORIENTED_EDGE('',*,*,#8420,.F.);
#11888=ORIENTED_EDGE('',*,*,#8421,.F.);
#11889=ORIENTED_EDGE('',*,*,#8349,.F.);
#11890=ORIENTED_EDGE('',*,*,#8422,.T.);
#11891=ORIENTED_EDGE('',*,*,#8423,.T.);
#11892=ORIENTED_EDGE('',*,*,#8424,.F.);
#11893=ORIENTED_EDGE('',*,*,#8385,.T.);
#11894=ORIENTED_EDGE('',*,*,#8425,.F.);
#11895=ORIENTED_EDGE('',*,*,#8426,.T.);
#11896=ORIENTED_EDGE('',*,*,#8427,.F.);
#11897=ORIENTED_EDGE('',*,*,#8381,.T.);
#11898=ORIENTED_EDGE('',*,*,#8428,.F.);
#11899=ORIENTED_EDGE('',*,*,#8429,.T.);
#11900=ORIENTED_EDGE('',*,*,#8430,.F.);
#11901=ORIENTED_EDGE('',*,*,#8377,.T.);
#11902=ORIENTED_EDGE('',*,*,#8431,.F.);
#11903=ORIENTED_EDGE('',*,*,#8432,.T.);
#11904=ORIENTED_EDGE('',*,*,#8433,.F.);
#11905=ORIENTED_EDGE('',*,*,#8373,.T.);
#11906=ORIENTED_EDGE('',*,*,#8434,.F.);
#11907=ORIENTED_EDGE('',*,*,#8435,.T.);
#11908=ORIENTED_EDGE('',*,*,#8436,.F.);
#11909=ORIENTED_EDGE('',*,*,#8369,.T.);
#11910=ORIENTED_EDGE('',*,*,#8437,.F.);
#11911=ORIENTED_EDGE('',*,*,#8438,.T.);
#11912=ORIENTED_EDGE('',*,*,#8439,.F.);
#11913=ORIENTED_EDGE('',*,*,#8365,.T.);
#11914=ORIENTED_EDGE('',*,*,#8440,.F.);
#11915=ORIENTED_EDGE('',*,*,#8441,.T.);
#11916=ORIENTED_EDGE('',*,*,#8442,.F.);
#11917=ORIENTED_EDGE('',*,*,#8361,.T.);
#11918=ORIENTED_EDGE('',*,*,#8443,.F.);
#11919=ORIENTED_EDGE('',*,*,#8355,.T.);
#11920=ORIENTED_EDGE('',*,*,#8350,.F.);
#11921=ORIENTED_EDGE('',*,*,#8444,.T.);
#11922=ORIENTED_EDGE('',*,*,#8445,.F.);
#11923=ORIENTED_EDGE('',*,*,#8420,.T.);
#11924=ORIENTED_EDGE('',*,*,#8446,.F.);
#11925=ORIENTED_EDGE('',*,*,#8447,.T.);
#11926=ORIENTED_EDGE('',*,*,#8448,.F.);
#11927=ORIENTED_EDGE('',*,*,#8416,.T.);
#11928=ORIENTED_EDGE('',*,*,#8449,.F.);
#11929=ORIENTED_EDGE('',*,*,#8450,.T.);
#11930=ORIENTED_EDGE('',*,*,#8451,.F.);
#11931=ORIENTED_EDGE('',*,*,#8412,.T.);
#11932=ORIENTED_EDGE('',*,*,#8452,.F.);
#11933=ORIENTED_EDGE('',*,*,#8453,.T.);
#11934=ORIENTED_EDGE('',*,*,#8454,.F.);
#11935=ORIENTED_EDGE('',*,*,#8408,.T.);
#11936=ORIENTED_EDGE('',*,*,#8455,.F.);
#11937=ORIENTED_EDGE('',*,*,#8456,.T.);
#11938=ORIENTED_EDGE('',*,*,#8457,.F.);
#11939=ORIENTED_EDGE('',*,*,#8404,.T.);
#11940=ORIENTED_EDGE('',*,*,#8458,.F.);
#11941=ORIENTED_EDGE('',*,*,#8459,.T.);
#11942=ORIENTED_EDGE('',*,*,#8460,.F.);
#11943=ORIENTED_EDGE('',*,*,#8400,.T.);
#11944=ORIENTED_EDGE('',*,*,#8461,.F.);
#11945=ORIENTED_EDGE('',*,*,#8462,.T.);
#11946=ORIENTED_EDGE('',*,*,#8463,.F.);
#11947=ORIENTED_EDGE('',*,*,#8396,.T.);
#11948=ORIENTED_EDGE('',*,*,#8464,.F.);
#11949=ORIENTED_EDGE('',*,*,#8465,.T.);
#11950=ORIENTED_EDGE('',*,*,#8466,.F.);
#11951=ORIENTED_EDGE('',*,*,#8392,.T.);
#11952=ORIENTED_EDGE('',*,*,#8467,.F.);
#11953=ORIENTED_EDGE('',*,*,#8468,.T.);
#11954=ORIENTED_EDGE('',*,*,#8422,.F.);
#11955=ORIENTED_EDGE('',*,*,#8445,.T.);
#11956=ORIENTED_EDGE('',*,*,#8469,.T.);
#11957=ORIENTED_EDGE('',*,*,#8470,.T.);
#11958=ORIENTED_EDGE('',*,*,#8421,.T.);
#11959=ORIENTED_EDGE('',*,*,#8446,.T.);
#11960=ORIENTED_EDGE('',*,*,#8419,.T.);
#11961=ORIENTED_EDGE('',*,*,#8471,.T.);
#11962=ORIENTED_EDGE('',*,*,#8472,.T.);
#11963=ORIENTED_EDGE('',*,*,#8448,.T.);
#11964=ORIENTED_EDGE('',*,*,#8473,.T.);
#11965=ORIENTED_EDGE('',*,*,#8474,.T.);
#11966=ORIENTED_EDGE('',*,*,#8417,.T.);
#11967=ORIENTED_EDGE('',*,*,#8449,.T.);
#11968=ORIENTED_EDGE('',*,*,#8415,.T.);
#11969=ORIENTED_EDGE('',*,*,#8475,.T.);
#11970=ORIENTED_EDGE('',*,*,#8476,.T.);
#11971=ORIENTED_EDGE('',*,*,#8451,.T.);
#11972=ORIENTED_EDGE('',*,*,#8477,.T.);
#11973=ORIENTED_EDGE('',*,*,#8478,.T.);
#11974=ORIENTED_EDGE('',*,*,#8413,.T.);
#11975=ORIENTED_EDGE('',*,*,#8452,.T.);
#11976=ORIENTED_EDGE('',*,*,#8411,.T.);
#11977=ORIENTED_EDGE('',*,*,#8479,.T.);
#11978=ORIENTED_EDGE('',*,*,#8480,.T.);
#11979=ORIENTED_EDGE('',*,*,#8454,.T.);
#11980=ORIENTED_EDGE('',*,*,#8481,.T.);
#11981=ORIENTED_EDGE('',*,*,#8482,.T.);
#11982=ORIENTED_EDGE('',*,*,#8409,.T.);
#11983=ORIENTED_EDGE('',*,*,#8455,.T.);
#11984=ORIENTED_EDGE('',*,*,#8407,.T.);
#11985=ORIENTED_EDGE('',*,*,#8483,.T.);
#11986=ORIENTED_EDGE('',*,*,#8484,.T.);
#11987=ORIENTED_EDGE('',*,*,#8457,.T.);
#11988=ORIENTED_EDGE('',*,*,#8485,.T.);
#11989=ORIENTED_EDGE('',*,*,#8486,.T.);
#11990=ORIENTED_EDGE('',*,*,#8405,.T.);
#11991=ORIENTED_EDGE('',*,*,#8458,.T.);
#11992=ORIENTED_EDGE('',*,*,#8403,.T.);
#11993=ORIENTED_EDGE('',*,*,#8487,.T.);
#11994=ORIENTED_EDGE('',*,*,#8488,.T.);
#11995=ORIENTED_EDGE('',*,*,#8460,.T.);
#11996=ORIENTED_EDGE('',*,*,#8489,.T.);
#11997=ORIENTED_EDGE('',*,*,#8490,.T.);
#11998=ORIENTED_EDGE('',*,*,#8401,.T.);
#11999=ORIENTED_EDGE('',*,*,#8461,.T.);
#12000=ORIENTED_EDGE('',*,*,#8399,.T.);
#12001=ORIENTED_EDGE('',*,*,#8491,.T.);
#12002=ORIENTED_EDGE('',*,*,#8492,.T.);
#12003=ORIENTED_EDGE('',*,*,#8463,.T.);
#12004=ORIENTED_EDGE('',*,*,#8493,.T.);
#12005=ORIENTED_EDGE('',*,*,#8494,.T.);
#12006=ORIENTED_EDGE('',*,*,#8397,.T.);
#12007=ORIENTED_EDGE('',*,*,#8464,.T.);
#12008=ORIENTED_EDGE('',*,*,#8395,.T.);
#12009=ORIENTED_EDGE('',*,*,#8495,.T.);
#12010=ORIENTED_EDGE('',*,*,#8496,.T.);
#12011=ORIENTED_EDGE('',*,*,#8466,.T.);
#12012=ORIENTED_EDGE('',*,*,#8497,.T.);
#12013=ORIENTED_EDGE('',*,*,#8498,.T.);
#12014=ORIENTED_EDGE('',*,*,#8393,.T.);
#12015=ORIENTED_EDGE('',*,*,#8467,.T.);
#12016=ORIENTED_EDGE('',*,*,#8391,.T.);
#12017=ORIENTED_EDGE('',*,*,#8499,.T.);
#12018=ORIENTED_EDGE('',*,*,#8500,.T.);
#12019=ORIENTED_EDGE('',*,*,#8424,.T.);
#12020=ORIENTED_EDGE('',*,*,#8501,.T.);
#12021=ORIENTED_EDGE('',*,*,#8502,.T.);
#12022=ORIENTED_EDGE('',*,*,#8386,.T.);
#12023=ORIENTED_EDGE('',*,*,#8425,.T.);
#12024=ORIENTED_EDGE('',*,*,#8384,.T.);
#12025=ORIENTED_EDGE('',*,*,#8503,.T.);
#12026=ORIENTED_EDGE('',*,*,#8504,.T.);
#12027=ORIENTED_EDGE('',*,*,#8427,.T.);
#12028=ORIENTED_EDGE('',*,*,#8505,.T.);
#12029=ORIENTED_EDGE('',*,*,#8506,.T.);
#12030=ORIENTED_EDGE('',*,*,#8382,.T.);
#12031=ORIENTED_EDGE('',*,*,#8428,.T.);
#12032=ORIENTED_EDGE('',*,*,#8380,.T.);
#12033=ORIENTED_EDGE('',*,*,#8507,.T.);
#12034=ORIENTED_EDGE('',*,*,#8508,.T.);
#12035=ORIENTED_EDGE('',*,*,#8430,.T.);
#12036=ORIENTED_EDGE('',*,*,#8509,.T.);
#12037=ORIENTED_EDGE('',*,*,#8510,.T.);
#12038=ORIENTED_EDGE('',*,*,#8378,.T.);
#12039=ORIENTED_EDGE('',*,*,#8431,.T.);
#12040=ORIENTED_EDGE('',*,*,#8376,.T.);
#12041=ORIENTED_EDGE('',*,*,#8511,.T.);
#12042=ORIENTED_EDGE('',*,*,#8512,.T.);
#12043=ORIENTED_EDGE('',*,*,#8433,.T.);
#12044=ORIENTED_EDGE('',*,*,#8513,.T.);
#12045=ORIENTED_EDGE('',*,*,#8514,.T.);
#12046=ORIENTED_EDGE('',*,*,#8374,.T.);
#12047=ORIENTED_EDGE('',*,*,#8434,.T.);
#12048=ORIENTED_EDGE('',*,*,#8372,.T.);
#12049=ORIENTED_EDGE('',*,*,#8515,.T.);
#12050=ORIENTED_EDGE('',*,*,#8516,.T.);
#12051=ORIENTED_EDGE('',*,*,#8436,.T.);
#12052=ORIENTED_EDGE('',*,*,#8517,.T.);
#12053=ORIENTED_EDGE('',*,*,#8518,.T.);
#12054=ORIENTED_EDGE('',*,*,#8370,.T.);
#12055=ORIENTED_EDGE('',*,*,#8437,.T.);
#12056=ORIENTED_EDGE('',*,*,#8368,.T.);
#12057=ORIENTED_EDGE('',*,*,#8519,.T.);
#12058=ORIENTED_EDGE('',*,*,#8520,.T.);
#12059=ORIENTED_EDGE('',*,*,#8439,.T.);
#12060=ORIENTED_EDGE('',*,*,#8521,.T.);
#12061=ORIENTED_EDGE('',*,*,#8522,.T.);
#12062=ORIENTED_EDGE('',*,*,#8366,.T.);
#12063=ORIENTED_EDGE('',*,*,#8440,.T.);
#12064=ORIENTED_EDGE('',*,*,#8364,.T.);
#12065=ORIENTED_EDGE('',*,*,#8523,.T.);
#12066=ORIENTED_EDGE('',*,*,#8524,.T.);
#12067=ORIENTED_EDGE('',*,*,#8442,.T.);
#12068=ORIENTED_EDGE('',*,*,#8525,.T.);
#12069=ORIENTED_EDGE('',*,*,#8526,.T.);
#12070=ORIENTED_EDGE('',*,*,#8362,.T.);
#12071=ORIENTED_EDGE('',*,*,#8527,.T.);
#12072=ORIENTED_EDGE('',*,*,#8528,.T.);
#12073=ORIENTED_EDGE('',*,*,#8356,.T.);
#12074=ORIENTED_EDGE('',*,*,#8443,.T.);
#12075=ORIENTED_EDGE('',*,*,#8360,.T.);
#12076=ORIENTED_EDGE('',*,*,#8529,.T.);
#12077=ORIENTED_EDGE('',*,*,#8530,.T.);
#12078=ORIENTED_EDGE('',*,*,#8531,.T.);
#12079=ORIENTED_EDGE('',*,*,#8357,.T.);
#12080=ORIENTED_EDGE('',*,*,#8528,.F.);
#12081=ORIENTED_EDGE('',*,*,#8359,.T.);
#12082=ORIENTED_EDGE('',*,*,#8532,.T.);
#12083=ORIENTED_EDGE('',*,*,#8533,.T.);
#12084=ORIENTED_EDGE('',*,*,#8529,.F.);
#12085=ORIENTED_EDGE('',*,*,#8530,.F.);
#12086=ORIENTED_EDGE('',*,*,#8527,.F.);
#12087=ORIENTED_EDGE('',*,*,#8533,.F.);
#12088=ORIENTED_EDGE('',*,*,#8534,.F.);
#12089=ORIENTED_EDGE('',*,*,#8348,.T.);
#12090=ORIENTED_EDGE('',*,*,#8535,.T.);
#12091=ORIENTED_EDGE('',*,*,#8536,.T.);
#12092=ORIENTED_EDGE('',*,*,#8535,.F.);
#12093=ORIENTED_EDGE('',*,*,#8537,.F.);
#12094=ORIENTED_EDGE('',*,*,#8538,.F.);
#12095=ORIENTED_EDGE('',*,*,#8539,.F.);
#12096=ORIENTED_EDGE('',*,*,#8540,.F.);
#12097=ORIENTED_EDGE('',*,*,#8541,.F.);
#12098=ORIENTED_EDGE('',*,*,#8542,.F.);
#12099=ORIENTED_EDGE('',*,*,#8536,.F.);
#12100=ORIENTED_EDGE('',*,*,#8543,.T.);
#12101=ORIENTED_EDGE('',*,*,#8544,.T.);
#12102=ORIENTED_EDGE('',*,*,#8545,.T.);
#12103=ORIENTED_EDGE('',*,*,#8546,.F.);
#12104=ORIENTED_EDGE('',*,*,#8547,.T.);
#12105=ORIENTED_EDGE('',*,*,#8548,.T.);
#12106=ORIENTED_EDGE('',*,*,#8549,.T.);
#12107=ORIENTED_EDGE('',*,*,#8544,.F.);
#12108=ORIENTED_EDGE('',*,*,#8550,.T.);
#12109=ORIENTED_EDGE('',*,*,#8551,.T.);
#12110=ORIENTED_EDGE('',*,*,#8552,.T.);
#12111=ORIENTED_EDGE('',*,*,#8553,.T.);
#12112=ORIENTED_EDGE('',*,*,#8554,.T.);
#12113=ORIENTED_EDGE('',*,*,#8551,.F.);
#12114=ORIENTED_EDGE('',*,*,#8555,.T.);
#12115=ORIENTED_EDGE('',*,*,#8556,.T.);
#12116=ORIENTED_EDGE('',*,*,#8557,.T.);
#12117=ORIENTED_EDGE('',*,*,#8553,.F.);
#12118=ORIENTED_EDGE('',*,*,#8558,.T.);
#12119=ORIENTED_EDGE('',*,*,#8548,.F.);
#12120=ORIENTED_EDGE('',*,*,#8559,.T.);
#12121=ORIENTED_EDGE('',*,*,#8556,.F.);
#12122=ORIENTED_EDGE('',*,*,#8560,.T.);
#12123=ORIENTED_EDGE('',*,*,#8546,.T.);
#12124=ORIENTED_EDGE('',*,*,#8549,.F.);
#12125=ORIENTED_EDGE('',*,*,#8561,.T.);
#12126=ORIENTED_EDGE('',*,*,#8542,.T.);
#12127=ORIENTED_EDGE('',*,*,#8562,.F.);
#12128=ORIENTED_EDGE('',*,*,#8558,.F.);
#12129=ORIENTED_EDGE('',*,*,#8563,.T.);
#12130=ORIENTED_EDGE('',*,*,#8537,.T.);
#12131=ORIENTED_EDGE('',*,*,#8561,.F.);
#12132=ORIENTED_EDGE('',*,*,#8552,.F.);
#12133=ORIENTED_EDGE('',*,*,#8564,.T.);
#12134=ORIENTED_EDGE('',*,*,#8538,.T.);
#12135=ORIENTED_EDGE('',*,*,#8563,.F.);
#12136=ORIENTED_EDGE('',*,*,#8565,.F.);
#12137=ORIENTED_EDGE('',*,*,#8550,.F.);
#12138=ORIENTED_EDGE('',*,*,#8557,.F.);
#12139=ORIENTED_EDGE('',*,*,#8547,.F.);
#12140=ORIENTED_EDGE('',*,*,#8543,.F.);
#12141=ORIENTED_EDGE('',*,*,#8560,.F.);
#12142=ORIENTED_EDGE('',*,*,#8555,.F.);
#12143=ORIENTED_EDGE('',*,*,#8554,.F.);
#12144=ORIENTED_EDGE('',*,*,#8566,.T.);
#12145=ORIENTED_EDGE('',*,*,#8539,.T.);
#12146=ORIENTED_EDGE('',*,*,#8564,.F.);
#12147=ORIENTED_EDGE('',*,*,#8559,.F.);
#12148=ORIENTED_EDGE('',*,*,#8567,.T.);
#12149=ORIENTED_EDGE('',*,*,#8540,.T.);
#12150=ORIENTED_EDGE('',*,*,#8566,.F.);
#12151=ORIENTED_EDGE('',*,*,#8545,.F.);
#12152=ORIENTED_EDGE('',*,*,#8562,.T.);
#12153=ORIENTED_EDGE('',*,*,#8541,.T.);
#12154=ORIENTED_EDGE('',*,*,#8567,.F.);
#12155=ORIENTED_EDGE('',*,*,#8358,.F.);
#12156=ORIENTED_EDGE('',*,*,#8531,.F.);
#12157=ORIENTED_EDGE('',*,*,#8534,.T.);
#12158=ORIENTED_EDGE('',*,*,#8532,.F.);
#12159=ORIENTED_EDGE('',*,*,#8524,.F.);
#12160=ORIENTED_EDGE('',*,*,#8568,.F.);
#12161=ORIENTED_EDGE('',*,*,#8525,.F.);
#12162=ORIENTED_EDGE('',*,*,#8441,.F.);
#12163=ORIENTED_EDGE('',*,*,#8363,.F.);
#12164=ORIENTED_EDGE('',*,*,#8526,.F.);
#12165=ORIENTED_EDGE('',*,*,#8568,.T.);
#12166=ORIENTED_EDGE('',*,*,#8523,.F.);
#12167=ORIENTED_EDGE('',*,*,#8367,.F.);
#12168=ORIENTED_EDGE('',*,*,#8522,.F.);
#12169=ORIENTED_EDGE('',*,*,#8569,.T.);
#12170=ORIENTED_EDGE('',*,*,#8519,.F.);
#12171=ORIENTED_EDGE('',*,*,#8520,.F.);
#12172=ORIENTED_EDGE('',*,*,#8569,.F.);
#12173=ORIENTED_EDGE('',*,*,#8521,.F.);
#12174=ORIENTED_EDGE('',*,*,#8438,.F.);
#12175=ORIENTED_EDGE('',*,*,#8516,.F.);
#12176=ORIENTED_EDGE('',*,*,#8570,.F.);
#12177=ORIENTED_EDGE('',*,*,#8517,.F.);
#12178=ORIENTED_EDGE('',*,*,#8435,.F.);
#12179=ORIENTED_EDGE('',*,*,#8371,.F.);
#12180=ORIENTED_EDGE('',*,*,#8518,.F.);
#12181=ORIENTED_EDGE('',*,*,#8570,.T.);
#12182=ORIENTED_EDGE('',*,*,#8515,.F.);
#12183=ORIENTED_EDGE('',*,*,#8375,.F.);
#12184=ORIENTED_EDGE('',*,*,#8514,.F.);
#12185=ORIENTED_EDGE('',*,*,#8571,.T.);
#12186=ORIENTED_EDGE('',*,*,#8511,.F.);
#12187=ORIENTED_EDGE('',*,*,#8512,.F.);
#12188=ORIENTED_EDGE('',*,*,#8571,.F.);
#12189=ORIENTED_EDGE('',*,*,#8513,.F.);
#12190=ORIENTED_EDGE('',*,*,#8432,.F.);
#12191=ORIENTED_EDGE('',*,*,#8508,.F.);
#12192=ORIENTED_EDGE('',*,*,#8572,.F.);
#12193=ORIENTED_EDGE('',*,*,#8509,.F.);
#12194=ORIENTED_EDGE('',*,*,#8429,.F.);
#12195=ORIENTED_EDGE('',*,*,#8379,.F.);
#12196=ORIENTED_EDGE('',*,*,#8510,.F.);
#12197=ORIENTED_EDGE('',*,*,#8572,.T.);
#12198=ORIENTED_EDGE('',*,*,#8507,.F.);
#12199=ORIENTED_EDGE('',*,*,#8383,.F.);
#12200=ORIENTED_EDGE('',*,*,#8506,.F.);
#12201=ORIENTED_EDGE('',*,*,#8573,.T.);
#12202=ORIENTED_EDGE('',*,*,#8503,.F.);
#12203=ORIENTED_EDGE('',*,*,#8504,.F.);
#12204=ORIENTED_EDGE('',*,*,#8573,.F.);
#12205=ORIENTED_EDGE('',*,*,#8505,.F.);
#12206=ORIENTED_EDGE('',*,*,#8426,.F.);
#12207=ORIENTED_EDGE('',*,*,#8500,.F.);
#12208=ORIENTED_EDGE('',*,*,#8574,.F.);
#12209=ORIENTED_EDGE('',*,*,#8501,.F.);
#12210=ORIENTED_EDGE('',*,*,#8423,.F.);
#12211=ORIENTED_EDGE('',*,*,#8468,.F.);
#12212=ORIENTED_EDGE('',*,*,#8387,.F.);
#12213=ORIENTED_EDGE('',*,*,#8502,.F.);
#12214=ORIENTED_EDGE('',*,*,#8574,.T.);
#12215=ORIENTED_EDGE('',*,*,#8499,.F.);
#12216=ORIENTED_EDGE('',*,*,#8390,.F.);
#12217=ORIENTED_EDGE('',*,*,#8394,.F.);
#12218=ORIENTED_EDGE('',*,*,#8498,.F.);
#12219=ORIENTED_EDGE('',*,*,#8575,.T.);
#12220=ORIENTED_EDGE('',*,*,#8495,.F.);
#12221=ORIENTED_EDGE('',*,*,#8496,.F.);
#12222=ORIENTED_EDGE('',*,*,#8575,.F.);
#12223=ORIENTED_EDGE('',*,*,#8497,.F.);
#12224=ORIENTED_EDGE('',*,*,#8465,.F.);
#12225=ORIENTED_EDGE('',*,*,#8492,.F.);
#12226=ORIENTED_EDGE('',*,*,#8576,.F.);
#12227=ORIENTED_EDGE('',*,*,#8493,.F.);
#12228=ORIENTED_EDGE('',*,*,#8462,.F.);
#12229=ORIENTED_EDGE('',*,*,#8398,.F.);
#12230=ORIENTED_EDGE('',*,*,#8494,.F.);
#12231=ORIENTED_EDGE('',*,*,#8576,.T.);
#12232=ORIENTED_EDGE('',*,*,#8491,.F.);
#12233=ORIENTED_EDGE('',*,*,#8402,.F.);
#12234=ORIENTED_EDGE('',*,*,#8490,.F.);
#12235=ORIENTED_EDGE('',*,*,#8577,.T.);
#12236=ORIENTED_EDGE('',*,*,#8487,.F.);
#12237=ORIENTED_EDGE('',*,*,#8488,.F.);
#12238=ORIENTED_EDGE('',*,*,#8577,.F.);
#12239=ORIENTED_EDGE('',*,*,#8489,.F.);
#12240=ORIENTED_EDGE('',*,*,#8459,.F.);
#12241=ORIENTED_EDGE('',*,*,#8484,.F.);
#12242=ORIENTED_EDGE('',*,*,#8578,.F.);
#12243=ORIENTED_EDGE('',*,*,#8485,.F.);
#12244=ORIENTED_EDGE('',*,*,#8456,.F.);
#12245=ORIENTED_EDGE('',*,*,#8406,.F.);
#12246=ORIENTED_EDGE('',*,*,#8486,.F.);
#12247=ORIENTED_EDGE('',*,*,#8578,.T.);
#12248=ORIENTED_EDGE('',*,*,#8483,.F.);
#12249=ORIENTED_EDGE('',*,*,#8410,.F.);
#12250=ORIENTED_EDGE('',*,*,#8482,.F.);
#12251=ORIENTED_EDGE('',*,*,#8579,.T.);
#12252=ORIENTED_EDGE('',*,*,#8479,.F.);
#12253=ORIENTED_EDGE('',*,*,#8480,.F.);
#12254=ORIENTED_EDGE('',*,*,#8579,.F.);
#12255=ORIENTED_EDGE('',*,*,#8481,.F.);
#12256=ORIENTED_EDGE('',*,*,#8453,.F.);
#12257=ORIENTED_EDGE('',*,*,#8476,.F.);
#12258=ORIENTED_EDGE('',*,*,#8580,.F.);
#12259=ORIENTED_EDGE('',*,*,#8477,.F.);
#12260=ORIENTED_EDGE('',*,*,#8450,.F.);
#12261=ORIENTED_EDGE('',*,*,#8414,.F.);
#12262=ORIENTED_EDGE('',*,*,#8478,.F.);
#12263=ORIENTED_EDGE('',*,*,#8580,.T.);
#12264=ORIENTED_EDGE('',*,*,#8475,.F.);
#12265=ORIENTED_EDGE('',*,*,#8418,.F.);
#12266=ORIENTED_EDGE('',*,*,#8474,.F.);
#12267=ORIENTED_EDGE('',*,*,#8581,.T.);
#12268=ORIENTED_EDGE('',*,*,#8471,.F.);
#12269=ORIENTED_EDGE('',*,*,#8472,.F.);
#12270=ORIENTED_EDGE('',*,*,#8581,.F.);
#12271=ORIENTED_EDGE('',*,*,#8473,.F.);
#12272=ORIENTED_EDGE('',*,*,#8447,.F.);
#12273=ORIENTED_EDGE('',*,*,#8353,.F.);
#12274=ORIENTED_EDGE('',*,*,#8582,.F.);
#12275=ORIENTED_EDGE('',*,*,#8469,.F.);
#12276=ORIENTED_EDGE('',*,*,#8444,.F.);
#12277=ORIENTED_EDGE('',*,*,#8354,.F.);
#12278=ORIENTED_EDGE('',*,*,#8470,.F.);
#12279=ORIENTED_EDGE('',*,*,#8582,.T.);
#12280=ORIENTED_EDGE('',*,*,#8352,.F.);
#12281=ORIENTED_EDGE('',*,*,#8389,.F.);
#12282=ORIENTED_EDGE('',*,*,#8583,.T.);
#12283=ORIENTED_EDGE('',*,*,#8565,.T.);
#12284=ORIENTED_EDGE('',*,*,#8583,.F.);
#13827=PLANE('',#15712);
#13828=PLANE('',#15714);
#13829=PLANE('',#15751);
#13830=PLANE('',#15752);
#13831=PLANE('',#15753);
#13832=PLANE('',#15754);
#13833=PLANE('',#15755);
#13834=PLANE('',#15756);
#13835=PLANE('',#15757);
#13836=PLANE('',#15758);
#13837=PLANE('',#15759);
#13838=PLANE('',#15760);
#13839=PLANE('',#15761);
#13840=PLANE('',#15762);
#13841=PLANE('',#15763);
#13842=PLANE('',#15764);
#13843=PLANE('',#15765);
#13844=PLANE('',#15766);
#13845=PLANE('',#15767);
#13846=PLANE('',#15768);
#13847=PLANE('',#15769);
#13848=PLANE('',#15770);
#13849=PLANE('',#15771);
#13850=PLANE('',#15772);
#13851=PLANE('',#15773);
#13852=PLANE('',#15774);
#13853=PLANE('',#15775);
#13854=PLANE('',#15776);
#13855=PLANE('',#15777);
#13856=PLANE('',#15778);
#13857=PLANE('',#15779);
#13858=PLANE('',#15780);
#13859=PLANE('',#15781);
#13860=PLANE('',#15786);
#13861=PLANE('',#15787);
#13862=PLANE('',#15788);
#13863=PLANE('',#15789);
#13864=PLANE('',#15790);
#13865=PLANE('',#15791);
#13866=PLANE('',#15792);
#13867=PLANE('',#15793);
#13868=PLANE('',#15794);
#13869=PLANE('',#15795);
#13870=PLANE('',#15796);
#13871=PLANE('',#15798);
#13872=PLANE('',#15799);
#13873=PLANE('',#15800);
#13874=PLANE('',#15801);
#13875=PLANE('',#15804);
#13876=PLANE('',#15805);
#13877=PLANE('',#15810);
#13878=PLANE('',#15811);
#13879=PLANE('',#15816);
#13880=PLANE('',#15817);
#13881=PLANE('',#15822);
#13882=PLANE('',#15823);
#13883=PLANE('',#15828);
#13884=PLANE('',#15829);
#13885=PLANE('',#15834);
#13886=PLANE('',#15835);
#13887=PLANE('',#15840);
#13888=PLANE('',#15841);
#13889=PLANE('',#15846);
#14477=ADVANCED_FACE('',(#1909),#1352,.F.);
#14478=ADVANCED_FACE('',(#1910),#786,.F.);
#14479=ADVANCED_FACE('',(#1911,#678),#13827,.T.);
#14480=ADVANCED_FACE('',(#1912),#13828,.T.);
#14481=ADVANCED_FACE('',(#1913),#787,.T.);
#14482=ADVANCED_FACE('',(#1914),#1353,.T.);
#14483=ADVANCED_FACE('',(#1915),#13829,.T.);
#14484=ADVANCED_FACE('',(#1916),#13830,.T.);
#14485=ADVANCED_FACE('',(#1917),#13831,.T.);
#14486=ADVANCED_FACE('',(#1918),#13832,.T.);
#14487=ADVANCED_FACE('',(#1919),#13833,.T.);
#14488=ADVANCED_FACE('',(#1920),#13834,.T.);
#14489=ADVANCED_FACE('',(#1921),#13835,.T.);
#14490=ADVANCED_FACE('',(#1922),#13836,.T.);
#14491=ADVANCED_FACE('',(#1923),#13837,.T.);
#14492=ADVANCED_FACE('',(#1924),#13838,.T.);
#14493=ADVANCED_FACE('',(#1925),#13839,.T.);
#14494=ADVANCED_FACE('',(#1926),#13840,.T.);
#14495=ADVANCED_FACE('',(#1927),#13841,.T.);
#14496=ADVANCED_FACE('',(#1928),#13842,.T.);
#14497=ADVANCED_FACE('',(#1929),#13843,.T.);
#14498=ADVANCED_FACE('',(#1930),#13844,.T.);
#14499=ADVANCED_FACE('',(#1931),#13845,.T.);
#14500=ADVANCED_FACE('',(#1932),#13846,.T.);
#14501=ADVANCED_FACE('',(#1933),#13847,.T.);
#14502=ADVANCED_FACE('',(#1934),#13848,.T.);
#14503=ADVANCED_FACE('',(#1935),#13849,.T.);
#14504=ADVANCED_FACE('',(#1936),#13850,.T.);
#14505=ADVANCED_FACE('',(#1937),#13851,.T.);
#14506=ADVANCED_FACE('',(#1938),#13852,.T.);
#14507=ADVANCED_FACE('',(#1939),#13853,.T.);
#14508=ADVANCED_FACE('',(#1940),#13854,.T.);
#14509=ADVANCED_FACE('',(#1941),#13855,.T.);
#14510=ADVANCED_FACE('',(#1942),#13856,.T.);
#14511=ADVANCED_FACE('',(#1943),#13857,.T.);
#14512=ADVANCED_FACE('',(#1944),#113,.T.);
#14513=ADVANCED_FACE('',(#1945),#13858,.T.);
#14514=ADVANCED_FACE('',(#1946),#13859,.T.);
#14515=ADVANCED_FACE('',(#1947),#788,.F.);
#14516=ADVANCED_FACE('',(#1948),#1354,.F.);
#14517=ADVANCED_FACE('',(#1949,#679),#13860,.F.);
#14518=ADVANCED_FACE('',(#1950),#13861,.T.);
#14519=ADVANCED_FACE('',(#1951),#13862,.T.);
#14520=ADVANCED_FACE('',(#1952),#13863,.T.);
#14521=ADVANCED_FACE('',(#1953),#13864,.T.);
#14522=ADVANCED_FACE('',(#1954),#13865,.T.);
#14523=ADVANCED_FACE('',(#1955),#13866,.T.);
#14524=ADVANCED_FACE('',(#1956),#13867,.F.);
#14525=ADVANCED_FACE('',(#1957),#13868,.F.);
#14526=ADVANCED_FACE('',(#1958),#13869,.F.);
#14527=ADVANCED_FACE('',(#1959,#680),#13870,.T.);
#14528=ADVANCED_FACE('',(#1960),#13871,.F.);
#14529=ADVANCED_FACE('',(#1961),#13872,.F.);
#14530=ADVANCED_FACE('',(#1962),#13873,.F.);
#14531=ADVANCED_FACE('',(#1963),#13874,.T.);
#14532=ADVANCED_FACE('',(#1964),#789,.F.);
#14533=ADVANCED_FACE('',(#1965),#13875,.T.);
#14534=ADVANCED_FACE('',(#1966),#13876,.T.);
#14535=ADVANCED_FACE('',(#1967),#790,.F.);
#14536=ADVANCED_FACE('',(#1968),#791,.F.);
#14537=ADVANCED_FACE('',(#1969),#13877,.T.);
#14538=ADVANCED_FACE('',(#1970),#13878,.T.);
#14539=ADVANCED_FACE('',(#1971),#792,.F.);
#14540=ADVANCED_FACE('',(#1972),#793,.F.);
#14541=ADVANCED_FACE('',(#1973),#13879,.T.);
#14542=ADVANCED_FACE('',(#1974),#13880,.T.);
#14543=ADVANCED_FACE('',(#1975),#794,.F.);
#14544=ADVANCED_FACE('',(#1976),#795,.F.);
#14545=ADVANCED_FACE('',(#1977),#13881,.T.);
#14546=ADVANCED_FACE('',(#1978),#13882,.T.);
#14547=ADVANCED_FACE('',(#1979),#796,.F.);
#14548=ADVANCED_FACE('',(#1980),#797,.F.);
#14549=ADVANCED_FACE('',(#1981),#13883,.T.);
#14550=ADVANCED_FACE('',(#1982),#13884,.T.);
#14551=ADVANCED_FACE('',(#1983),#798,.F.);
#14552=ADVANCED_FACE('',(#1984),#799,.F.);
#14553=ADVANCED_FACE('',(#1985),#13885,.T.);
#14554=ADVANCED_FACE('',(#1986),#13886,.T.);
#14555=ADVANCED_FACE('',(#1987),#800,.F.);
#14556=ADVANCED_FACE('',(#1988),#801,.F.);
#14557=ADVANCED_FACE('',(#1989),#13887,.T.);
#14558=ADVANCED_FACE('',(#1990),#13888,.T.);
#14559=ADVANCED_FACE('',(#1991),#802,.F.);
#14560=ADVANCED_FACE('',(#1992),#803,.F.);
#14561=ADVANCED_FACE('',(#1993),#13889,.T.);
#14562=ADVANCED_FACE('',(#1994),#1355,.T.);
#14783=CLOSED_SHELL('',(#14477,#14478,#14479,#14480,#14481,#14482,#14483,
#14484,#14485,#14486,#14487,#14488,#14489,#14490,#14491,#14492,#14493,#14494,
#14495,#14496,#14497,#14498,#14499,#14500,#14501,#14502,#14503,#14504,#14505,
#14506,#14507,#14508,#14509,#14510,#14511,#14512,#14513,#14514,#14515,#14516,
#14517,#14518,#14519,#14520,#14521,#14522,#14523,#14524,#14525,#14526,#14527,
#14528,#14529,#14530,#14531,#14532,#14533,#14534,#14535,#14536,#14537,#14538,
#14539,#14540,#14541,#14542,#14543,#14544,#14545,#14546,#14547,#14548,#14549,
#14550,#14551,#14552,#14553,#14554,#14555,#14556,#14557,#14558,#14559,#14560,
#14561,#14562));
#15705=AXIS2_PLACEMENT_3D('',#26207,#18575,#18576);
#15706=AXIS2_PLACEMENT_3D('',#26208,#18577,#18578);
#15707=AXIS2_PLACEMENT_3D('',#26211,#18579,#18580);
#15708=AXIS2_PLACEMENT_3D('',#26212,#18581,#18582);
#15709=AXIS2_PLACEMENT_3D('',#26215,#18584,#18585);
#15710=AXIS2_PLACEMENT_3D('',#26216,#18586,#18587);
#15711=AXIS2_PLACEMENT_3D('',#26219,#18589,#18590);
#15712=AXIS2_PLACEMENT_3D('',#26220,#18591,#18592);
#15713=AXIS2_PLACEMENT_3D('',#26222,#18593,#18594);
#15714=AXIS2_PLACEMENT_3D('',#26223,#18595,#18596);
#15715=AXIS2_PLACEMENT_3D('',#26234,#18600,#18601);
#15716=AXIS2_PLACEMENT_3D('',#26236,#18602,#18603);
#15717=AXIS2_PLACEMENT_3D('',#26238,#18604,#18605);
#15718=AXIS2_PLACEMENT_3D('',#26247,#18607,#18608);
#15719=AXIS2_PLACEMENT_3D('',#26256,#18610,#18611);
#15720=AXIS2_PLACEMENT_3D('',#26260,#18613,#18614);
#15721=AXIS2_PLACEMENT_3D('',#26264,#18616,#18617);
#15722=AXIS2_PLACEMENT_3D('',#26268,#18619,#18620);
#15723=AXIS2_PLACEMENT_3D('',#26272,#18622,#18623);
#15724=AXIS2_PLACEMENT_3D('',#26276,#18625,#18626);
#15725=AXIS2_PLACEMENT_3D('',#26280,#18628,#18629);
#15726=AXIS2_PLACEMENT_3D('',#26284,#18631,#18632);
#15727=AXIS2_PLACEMENT_3D('',#26288,#18634,#18635);
#15728=AXIS2_PLACEMENT_3D('',#26292,#18637,#18638);
#15729=AXIS2_PLACEMENT_3D('',#26296,#18640,#18641);
#15730=AXIS2_PLACEMENT_3D('',#26300,#18643,#18644);
#15731=AXIS2_PLACEMENT_3D('',#26304,#18646,#18647);
#15732=AXIS2_PLACEMENT_3D('',#26308,#18649,#18650);
#15733=AXIS2_PLACEMENT_3D('',#26311,#18652,#18653);
#15734=AXIS2_PLACEMENT_3D('',#26313,#18654,#18655);
#15735=AXIS2_PLACEMENT_3D('',#26317,#18657,#18658);
#15736=AXIS2_PLACEMENT_3D('',#26321,#18660,#18661);
#15737=AXIS2_PLACEMENT_3D('',#26325,#18663,#18664);
#15738=AXIS2_PLACEMENT_3D('',#26329,#18666,#18667);
#15739=AXIS2_PLACEMENT_3D('',#26333,#18669,#18670);
#15740=AXIS2_PLACEMENT_3D('',#26337,#18672,#18673);
#15741=AXIS2_PLACEMENT_3D('',#26341,#18675,#18676);
#15742=AXIS2_PLACEMENT_3D('',#26345,#18678,#18679);
#15743=AXIS2_PLACEMENT_3D('',#26349,#18681,#18682);
#15744=AXIS2_PLACEMENT_3D('',#26353,#18684,#18685);
#15745=AXIS2_PLACEMENT_3D('',#26357,#18687,#18688);
#15746=AXIS2_PLACEMENT_3D('',#26361,#18690,#18691);
#15747=AXIS2_PLACEMENT_3D('',#26365,#18693,#18694);
#15748=AXIS2_PLACEMENT_3D('',#26369,#18696,#18697);
#15749=AXIS2_PLACEMENT_3D('',#26373,#18699,#18700);
#15750=AXIS2_PLACEMENT_3D('',#26375,#18702,#18703);
#15751=AXIS2_PLACEMENT_3D('',#26655,#18705,#18706);
#15752=AXIS2_PLACEMENT_3D('',#26659,#18709,#18710);
#15753=AXIS2_PLACEMENT_3D('',#26663,#18713,#18714);
#15754=AXIS2_PLACEMENT_3D('',#26667,#18717,#18718);
#15755=AXIS2_PLACEMENT_3D('',#26671,#18721,#18722);
#15756=AXIS2_PLACEMENT_3D('',#26675,#18725,#18726);
#15757=AXIS2_PLACEMENT_3D('',#26679,#18729,#18730);
#15758=AXIS2_PLACEMENT_3D('',#26683,#18733,#18734);
#15759=AXIS2_PLACEMENT_3D('',#26687,#18737,#18738);
#15760=AXIS2_PLACEMENT_3D('',#26691,#18741,#18742);
#15761=AXIS2_PLACEMENT_3D('',#26695,#18745,#18746);
#15762=AXIS2_PLACEMENT_3D('',#26699,#18749,#18750);
#15763=AXIS2_PLACEMENT_3D('',#26703,#18753,#18754);
#15764=AXIS2_PLACEMENT_3D('',#26707,#18757,#18758);
#15765=AXIS2_PLACEMENT_3D('',#26711,#18761,#18762);
#15766=AXIS2_PLACEMENT_3D('',#26715,#18765,#18766);
#15767=AXIS2_PLACEMENT_3D('',#26719,#18769,#18770);
#15768=AXIS2_PLACEMENT_3D('',#26723,#18773,#18774);
#15769=AXIS2_PLACEMENT_3D('',#26727,#18777,#18778);
#15770=AXIS2_PLACEMENT_3D('',#26731,#18781,#18782);
#15771=AXIS2_PLACEMENT_3D('',#26735,#18785,#18786);
#15772=AXIS2_PLACEMENT_3D('',#26739,#18789,#18790);
#15773=AXIS2_PLACEMENT_3D('',#26743,#18793,#18794);
#15774=AXIS2_PLACEMENT_3D('',#26747,#18797,#18798);
#15775=AXIS2_PLACEMENT_3D('',#26751,#18801,#18802);
#15776=AXIS2_PLACEMENT_3D('',#26755,#18805,#18806);
#15777=AXIS2_PLACEMENT_3D('',#26759,#18809,#18810);
#15778=AXIS2_PLACEMENT_3D('',#26763,#18813,#18814);
#15779=AXIS2_PLACEMENT_3D('',#26767,#18817,#18818);
#15780=AXIS2_PLACEMENT_3D('',#26851,#18821,#18822);
#15781=AXIS2_PLACEMENT_3D('',#26855,#18825,#18826);
#15782=AXIS2_PLACEMENT_3D('',#26859,#18829,#18830);
#15783=AXIS2_PLACEMENT_3D('',#26860,#18831,#18832);
#15784=AXIS2_PLACEMENT_3D('',#26861,#18833,#18834);
#15785=AXIS2_PLACEMENT_3D('',#26864,#18836,#18837);
#15786=AXIS2_PLACEMENT_3D('',#26865,#18838,#18839);
#15787=AXIS2_PLACEMENT_3D('',#26878,#18846,#18847);
#15788=AXIS2_PLACEMENT_3D('',#26887,#18852,#18853);
#15789=AXIS2_PLACEMENT_3D('',#26893,#18857,#18858);
#15790=AXIS2_PLACEMENT_3D('',#26902,#18863,#18864);
#15791=AXIS2_PLACEMENT_3D('',#26908,#18868,#18869);
#15792=AXIS2_PLACEMENT_3D('',#26911,#18872,#18873);
#15793=AXIS2_PLACEMENT_3D('',#26914,#18876,#18877);
#15794=AXIS2_PLACEMENT_3D('',#26917,#18880,#18881);
#15795=AXIS2_PLACEMENT_3D('',#26919,#18883,#18884);
#15796=AXIS2_PLACEMENT_3D('',#26921,#18886,#18887);
#15797=AXIS2_PLACEMENT_3D('',#26923,#18888,#18889);
#15798=AXIS2_PLACEMENT_3D('',#26924,#18890,#18891);
#15799=AXIS2_PLACEMENT_3D('',#26926,#18893,#18894);
#15800=AXIS2_PLACEMENT_3D('',#26928,#18896,#18897);
#15801=AXIS2_PLACEMENT_3D('',#26929,#18898,#18899);
#15802=AXIS2_PLACEMENT_3D('',#26930,#18900,#18901);
#15803=AXIS2_PLACEMENT_3D('',#26931,#18902,#18903);
#15804=AXIS2_PLACEMENT_3D('',#26932,#18904,#18905);
#15805=AXIS2_PLACEMENT_3D('',#26933,#18906,#18907);
#15806=AXIS2_PLACEMENT_3D('',#26934,#18908,#18909);
#15807=AXIS2_PLACEMENT_3D('',#26935,#18910,#18911);
#15808=AXIS2_PLACEMENT_3D('',#26936,#18912,#18913);
#15809=AXIS2_PLACEMENT_3D('',#26937,#18914,#18915);
#15810=AXIS2_PLACEMENT_3D('',#26938,#18916,#18917);
#15811=AXIS2_PLACEMENT_3D('',#26939,#18918,#18919);
#15812=AXIS2_PLACEMENT_3D('',#26940,#18920,#18921);
#15813=AXIS2_PLACEMENT_3D('',#26941,#18922,#18923);
#15814=AXIS2_PLACEMENT_3D('',#26942,#18924,#18925);
#15815=AXIS2_PLACEMENT_3D('',#26943,#18926,#18927);
#15816=AXIS2_PLACEMENT_3D('',#26944,#18928,#18929);
#15817=AXIS2_PLACEMENT_3D('',#26945,#18930,#18931);
#15818=AXIS2_PLACEMENT_3D('',#26946,#18932,#18933);
#15819=AXIS2_PLACEMENT_3D('',#26947,#18934,#18935);
#15820=AXIS2_PLACEMENT_3D('',#26948,#18936,#18937);
#15821=AXIS2_PLACEMENT_3D('',#26949,#18938,#18939);
#15822=AXIS2_PLACEMENT_3D('',#26950,#18940,#18941);
#15823=AXIS2_PLACEMENT_3D('',#26951,#18942,#18943);
#15824=AXIS2_PLACEMENT_3D('',#26952,#18944,#18945);
#15825=AXIS2_PLACEMENT_3D('',#26953,#18946,#18947);
#15826=AXIS2_PLACEMENT_3D('',#26954,#18948,#18949);
#15827=AXIS2_PLACEMENT_3D('',#26955,#18950,#18951);
#15828=AXIS2_PLACEMENT_3D('',#26956,#18952,#18953);
#15829=AXIS2_PLACEMENT_3D('',#26957,#18954,#18955);
#15830=AXIS2_PLACEMENT_3D('',#26958,#18956,#18957);
#15831=AXIS2_PLACEMENT_3D('',#26959,#18958,#18959);
#15832=AXIS2_PLACEMENT_3D('',#26960,#18960,#18961);
#15833=AXIS2_PLACEMENT_3D('',#26961,#18962,#18963);
#15834=AXIS2_PLACEMENT_3D('',#26962,#18964,#18965);
#15835=AXIS2_PLACEMENT_3D('',#26963,#18966,#18967);
#15836=AXIS2_PLACEMENT_3D('',#26964,#18968,#18969);
#15837=AXIS2_PLACEMENT_3D('',#26965,#18970,#18971);
#15838=AXIS2_PLACEMENT_3D('',#26966,#18972,#18973);
#15839=AXIS2_PLACEMENT_3D('',#26967,#18974,#18975);
#15840=AXIS2_PLACEMENT_3D('',#26968,#18976,#18977);
#15841=AXIS2_PLACEMENT_3D('',#26969,#18978,#18979);
#15842=AXIS2_PLACEMENT_3D('',#26970,#18980,#18981);
#15843=AXIS2_PLACEMENT_3D('',#26971,#18982,#18983);
#15844=AXIS2_PLACEMENT_3D('',#26972,#18984,#18985);
#15845=AXIS2_PLACEMENT_3D('',#26973,#18986,#18987);
#15846=AXIS2_PLACEMENT_3D('',#26974,#18988,#18989);
#15847=AXIS2_PLACEMENT_3D('',#26975,#18990,#18991);
#18575=DIRECTION('axis',(0.,0.,1.));
#18576=DIRECTION('refdir',(1.,0.,0.));
#18577=DIRECTION('center_axis',(1.,0.,0.));
#18578=DIRECTION('ref_axis',(0.,-1.,0.));
#18579=DIRECTION('center_axis',(-1.,0.,0.));
#18580=DIRECTION('ref_axis',(0.,-1.,0.));
#18581=DIRECTION('center_axis',(-1.,0.,0.));
#18582=DIRECTION('ref_axis',(0.,-1.,0.));
#18583=DIRECTION('',(0.707106781186548,0.707106781186547,-8.65956056235493E-17));
#18584=DIRECTION('center_axis',(1.,0.,0.));
#18585=DIRECTION('ref_axis',(0.,-1.,0.));
#18586=DIRECTION('center_axis',(1.,0.,0.));
#18587=DIRECTION('ref_axis',(0.,1.,0.));
#18588=DIRECTION('',(-1.,0.,0.));
#18589=DIRECTION('center_axis',(1.,0.,0.));
#18590=DIRECTION('ref_axis',(0.,1.,0.));
#18591=DIRECTION('center_axis',(1.,0.,0.));
#18592=DIRECTION('ref_axis',(0.,0.,-1.));
#18593=DIRECTION('center_axis',(1.,0.,0.));
#18594=DIRECTION('ref_axis',(0.,0.,-1.));
#18595=DIRECTION('center_axis',(0.,0.946649377085496,0.322265351633779));
#18596=DIRECTION('ref_axis',(0.,-0.322265351633779,0.946649377085496));
#18597=DIRECTION('',(-1.,0.,0.));
#18598=DIRECTION('',(0.,0.322265351633779,-0.946649377085496));
#18599=DIRECTION('',(1.,0.,0.));
#18600=DIRECTION('center_axis',(1.,0.,0.));
#18601=DIRECTION('ref_axis',(0.,1.,0.));
#18602=DIRECTION('center_axis',(-1.,0.,0.));
#18603=DIRECTION('ref_axis',(0.,1.,0.));
#18604=DIRECTION('center_axis',(1.,0.,0.));
#18605=DIRECTION('ref_axis',(0.,0.,-1.));
#18606=DIRECTION('',(1.,0.,0.));
#18607=DIRECTION('center_axis',(-1.,0.,0.));
#18608=DIRECTION('ref_axis',(0.,1.,0.));
#18609=DIRECTION('',(-1.,0.,0.));
#18610=DIRECTION('center_axis',(1.,0.,0.));
#18611=DIRECTION('ref_axis',(0.,0.,-1.));
#18612=DIRECTION('',(1.,0.,0.));
#18613=DIRECTION('center_axis',(-1.,0.,0.));
#18614=DIRECTION('ref_axis',(0.,1.,0.));
#18615=DIRECTION('',(-1.,0.,0.));
#18616=DIRECTION('center_axis',(1.,0.,0.));
#18617=DIRECTION('ref_axis',(0.,0.,-1.));
#18618=DIRECTION('',(1.,0.,0.));
#18619=DIRECTION('center_axis',(-1.,0.,0.));
#18620=DIRECTION('ref_axis',(0.,1.,0.));
#18621=DIRECTION('',(-1.,0.,0.));
#18622=DIRECTION('center_axis',(1.,0.,0.));
#18623=DIRECTION('ref_axis',(0.,0.,-1.));
#18624=DIRECTION('',(1.,0.,0.));
#18625=DIRECTION('center_axis',(-1.,0.,0.));
#18626=DIRECTION('ref_axis',(0.,1.,0.));
#18627=DIRECTION('',(-1.,0.,0.));
#18628=DIRECTION('center_axis',(1.,0.,0.));
#18629=DIRECTION('ref_axis',(0.,0.,-1.));
#18630=DIRECTION('',(1.,0.,0.));
#18631=DIRECTION('center_axis',(-1.,0.,0.));
#18632=DIRECTION('ref_axis',(0.,1.,0.));
#18633=DIRECTION('',(-1.,0.,0.));
#18634=DIRECTION('center_axis',(1.,0.,0.));
#18635=DIRECTION('ref_axis',(0.,0.,-1.));
#18636=DIRECTION('',(1.,0.,0.));
#18637=DIRECTION('center_axis',(-1.,0.,0.));
#18638=DIRECTION('ref_axis',(0.,1.,0.));
#18639=DIRECTION('',(-1.,0.,0.));
#18640=DIRECTION('center_axis',(1.,0.,0.));
#18641=DIRECTION('ref_axis',(0.,0.,-1.));
#18642=DIRECTION('',(1.,0.,0.));
#18643=DIRECTION('center_axis',(-1.,0.,0.));
#18644=DIRECTION('ref_axis',(0.,1.,0.));
#18645=DIRECTION('',(-1.,0.,0.));
#18646=DIRECTION('center_axis',(1.,0.,0.));
#18647=DIRECTION('ref_axis',(0.,0.,-1.));
#18648=DIRECTION('',(1.,0.,0.));
#18649=DIRECTION('center_axis',(-1.,0.,0.));
#18650=DIRECTION('ref_axis',(0.,1.,0.));
#18651=DIRECTION('',(-1.,0.,0.));
#18652=DIRECTION('center_axis',(1.,0.,0.));
#18653=DIRECTION('ref_axis',(0.,0.,-1.));
#18654=DIRECTION('center_axis',(-1.,0.,0.));
#18655=DIRECTION('ref_axis',(0.,1.,0.));
#18656=DIRECTION('',(-1.,0.,0.));
#18657=DIRECTION('center_axis',(1.,0.,0.));
#18658=DIRECTION('ref_axis',(0.,0.,-1.));
#18659=DIRECTION('',(1.,0.,0.));
#18660=DIRECTION('center_axis',(-1.,0.,0.));
#18661=DIRECTION('ref_axis',(0.,1.,0.));
#18662=DIRECTION('',(-1.,0.,0.));
#18663=DIRECTION('center_axis',(1.,0.,0.));
#18664=DIRECTION('ref_axis',(0.,0.,-1.));
#18665=DIRECTION('',(1.,0.,0.));
#18666=DIRECTION('center_axis',(-1.,0.,0.));
#18667=DIRECTION('ref_axis',(0.,1.,0.));
#18668=DIRECTION('',(-1.,0.,0.));
#18669=DIRECTION('center_axis',(1.,0.,0.));
#18670=DIRECTION('ref_axis',(0.,0.,-1.));
#18671=DIRECTION('',(1.,0.,0.));
#18672=DIRECTION('center_axis',(-1.,0.,0.));
#18673=DIRECTION('ref_axis',(0.,1.,0.));
#18674=DIRECTION('',(-1.,0.,0.));
#18675=DIRECTION('center_axis',(1.,0.,0.));
#18676=DIRECTION('ref_axis',(0.,0.,-1.));
#18677=DIRECTION('',(1.,0.,0.));
#18678=DIRECTION('center_axis',(-1.,0.,0.));
#18679=DIRECTION('ref_axis',(0.,1.,0.));
#18680=DIRECTION('',(-1.,0.,0.));
#18681=DIRECTION('center_axis',(1.,0.,0.));
#18682=DIRECTION('ref_axis',(0.,0.,-1.));
#18683=DIRECTION('',(1.,0.,0.));
#18684=DIRECTION('center_axis',(-1.,0.,0.));
#18685=DIRECTION('ref_axis',(0.,1.,0.));
#18686=DIRECTION('',(-1.,0.,0.));
#18687=DIRECTION('center_axis',(1.,0.,0.));
#18688=DIRECTION('ref_axis',(0.,0.,-1.));
#18689=DIRECTION('',(1.,0.,0.));
#18690=DIRECTION('center_axis',(-1.,0.,0.));
#18691=DIRECTION('ref_axis',(0.,1.,0.));
#18692=DIRECTION('',(-1.,0.,0.));
#18693=DIRECTION('center_axis',(1.,0.,0.));
#18694=DIRECTION('ref_axis',(0.,0.,-1.));
#18695=DIRECTION('',(1.,0.,0.));
#18696=DIRECTION('center_axis',(-1.,0.,0.));
#18697=DIRECTION('ref_axis',(0.,1.,0.));
#18698=DIRECTION('',(-1.,0.,0.));
#18699=DIRECTION('center_axis',(1.,0.,0.));
#18700=DIRECTION('ref_axis',(0.,0.,-1.));
#18701=DIRECTION('',(1.,0.,0.));
#18702=DIRECTION('center_axis',(-1.,0.,0.));
#18703=DIRECTION('ref_axis',(0.,1.,0.));
#18704=DIRECTION('',(-0.707106781186548,-0.707106781186547,-8.65956056235493E-17));
#18705=DIRECTION('center_axis',(0.,0.946649377085496,-0.322265351633779));
#18706=DIRECTION('ref_axis',(0.,0.322265351633779,0.946649377085496));
#18707=DIRECTION('',(-1.,0.,0.));
#18708=DIRECTION('',(0.,-0.322265351633779,-0.946649377085496));
#18709=DIRECTION('center_axis',(0.,0.751264373058291,0.660001395281354));
#18710=DIRECTION('ref_axis',(1.,0.,0.));
#18711=DIRECTION('',(0.,0.660001395281354,-0.751264373058291));
#18712=DIRECTION('',(1.,0.,0.));
#18713=DIRECTION('center_axis',(0.,0.997915594849406,0.0645326704573513));
#18714=DIRECTION('ref_axis',(0.,-0.0645326704573513,0.997915594849406));
#18715=DIRECTION('',(-1.,0.,0.));
#18716=DIRECTION('',(0.,0.0645326704573513,-0.997915594849406));
#18717=DIRECTION('center_axis',(0.,0.441506178461464,0.897258209424887));
#18718=DIRECTION('ref_axis',(1.,0.,0.));
#18719=DIRECTION('',(0.,0.897258209424887,-0.441506178461464));
#18720=DIRECTION('',(1.,0.,0.));
#18721=DIRECTION('center_axis',(0.,0.897258209424887,0.441506178461464));
#18722=DIRECTION('ref_axis',(0.,-0.441506178461464,0.897258209424887));
#18723=DIRECTION('',(-1.,0.,0.));
#18724=DIRECTION('',(0.,0.441506178461464,-0.897258209424887));
#18725=DIRECTION('center_axis',(0.,0.0645326704573477,0.997915594849406));
#18726=DIRECTION('ref_axis',(1.,0.,0.));
#18727=DIRECTION('',(0.,0.997915594849406,-0.0645326704573477));
#18728=DIRECTION('',(1.,0.,0.));
#18729=DIRECTION('center_axis',(0.,0.660001395281354,0.751264373058291));
#18730=DIRECTION('ref_axis',(1.,0.,0.));
#18731=DIRECTION('',(-1.,0.,0.));
#18732=DIRECTION('',(0.,0.751264373058291,-0.660001395281354));
#18733=DIRECTION('center_axis',(0.,-0.322265351633779,0.946649377085496));
#18734=DIRECTION('ref_axis',(1.,0.,0.));
#18735=DIRECTION('',(0.,0.946649377085496,0.322265351633779));
#18736=DIRECTION('',(1.,0.,0.));
#18737=DIRECTION('center_axis',(0.,0.322265351633779,0.946649377085496));
#18738=DIRECTION('ref_axis',(1.,0.,0.));
#18739=DIRECTION('',(-1.,0.,0.));
#18740=DIRECTION('',(0.,0.946649377085496,-0.322265351633779));
#18741=DIRECTION('center_axis',(0.,-0.660001395281353,0.751264373058291));
#18742=DIRECTION('ref_axis',(1.,0.,0.));
#18743=DIRECTION('',(0.,0.751264373058291,0.660001395281353));
#18744=DIRECTION('',(1.,0.,0.));
#18745=DIRECTION('center_axis',(0.,-0.0645326704573494,0.997915594849406));
#18746=DIRECTION('ref_axis',(1.,0.,0.));
#18747=DIRECTION('',(-1.,0.,0.));
#18748=DIRECTION('',(0.,0.997915594849406,0.0645326704573494));
#18749=DIRECTION('center_axis',(0.,-0.897258209424888,0.441506178461462));
#18750=DIRECTION('ref_axis',(0.,-0.441506178461462,-0.897258209424888));
#18751=DIRECTION('',(0.,0.441506178461462,0.897258209424888));
#18752=DIRECTION('',(1.,0.,0.));
#18753=DIRECTION('center_axis',(0.,-0.441506178461463,0.897258209424887));
#18754=DIRECTION('ref_axis',(1.,0.,0.));
#18755=DIRECTION('',(-1.,0.,0.));
#18756=DIRECTION('',(0.,0.897258209424887,0.441506178461463));
#18757=DIRECTION('center_axis',(0.,-0.997915594849406,0.0645326704573477));
#18758=DIRECTION('ref_axis',(0.,-0.0645326704573477,-0.997915594849406));
#18759=DIRECTION('',(0.,0.0645326704573477,0.997915594849406));
#18760=DIRECTION('',(1.,0.,0.));
#18761=DIRECTION('center_axis',(0.,-0.751264373058291,0.660001395281354));
#18762=DIRECTION('ref_axis',(1.,0.,0.));
#18763=DIRECTION('',(-1.,0.,0.));
#18764=DIRECTION('',(0.,0.660001395281354,0.751264373058291));
#18765=DIRECTION('center_axis',(0.,-0.946649377085496,-0.322265351633779));
#18766=DIRECTION('ref_axis',(0.,0.322265351633779,-0.946649377085496));
#18767=DIRECTION('',(0.,-0.322265351633779,0.946649377085496));
#18768=DIRECTION('',(1.,0.,0.));
#18769=DIRECTION('center_axis',(0.,-0.946649377085496,0.322265351633779));
#18770=DIRECTION('ref_axis',(0.,-0.322265351633779,-0.946649377085496));
#18771=DIRECTION('',(-1.,0.,0.));
#18772=DIRECTION('',(0.,0.322265351633779,0.946649377085496));
#18773=DIRECTION('center_axis',(0.,-0.75126437305829,-0.660001395281354));
#18774=DIRECTION('ref_axis',(-1.,0.,0.));
#18775=DIRECTION('',(0.,-0.660001395281354,0.75126437305829));
#18776=DIRECTION('',(1.,0.,0.));
#18777=DIRECTION('center_axis',(0.,-0.997915594849406,-0.0645326704573514));
#18778=DIRECTION('ref_axis',(0.,0.0645326704573514,-0.997915594849406));
#18779=DIRECTION('',(-1.,0.,0.));
#18780=DIRECTION('',(0.,-0.0645326704573514,0.997915594849406));
#18781=DIRECTION('center_axis',(0.,-0.441506178461457,-0.89725820942489));
#18782=DIRECTION('ref_axis',(-1.,0.,0.));
#18783=DIRECTION('',(0.,-0.89725820942489,0.441506178461457));
#18784=DIRECTION('',(1.,0.,0.));
#18785=DIRECTION('center_axis',(0.,-0.89725820942489,-0.441506178461457));
#18786=DIRECTION('ref_axis',(0.,0.441506178461457,-0.89725820942489));
#18787=DIRECTION('',(-1.,0.,0.));
#18788=DIRECTION('',(0.,-0.441506178461457,0.89725820942489));
#18789=DIRECTION('center_axis',(0.,-0.0645326704573515,-0.997915594849406));
#18790=DIRECTION('ref_axis',(-1.,0.,0.));
#18791=DIRECTION('',(0.,-0.997915594849406,0.0645326704573514));
#18792=DIRECTION('',(1.,0.,0.));
#18793=DIRECTION('center_axis',(0.,-0.660001395281353,-0.751264373058291));
#18794=DIRECTION('ref_axis',(-1.,0.,0.));
#18795=DIRECTION('',(-1.,0.,0.));
#18796=DIRECTION('',(0.,-0.751264373058291,0.660001395281353));
#18797=DIRECTION('center_axis',(0.,0.322265351633779,-0.946649377085496));
#18798=DIRECTION('ref_axis',(-1.,0.,0.));
#18799=DIRECTION('',(0.,-0.946649377085496,-0.322265351633779));
#18800=DIRECTION('',(1.,0.,0.));
#18801=DIRECTION('center_axis',(0.,-0.322265351633779,-0.946649377085496));
#18802=DIRECTION('ref_axis',(-1.,0.,0.));
#18803=DIRECTION('',(-1.,0.,0.));
#18804=DIRECTION('',(0.,-0.946649377085496,0.322265351633779));
#18805=DIRECTION('center_axis',(0.,0.660001395281352,-0.751264373058292));
#18806=DIRECTION('ref_axis',(-1.,0.,0.));
#18807=DIRECTION('',(0.,-0.751264373058292,-0.660001395281352));
#18808=DIRECTION('',(1.,0.,0.));
#18809=DIRECTION('center_axis',(0.,0.0645326704573514,-0.997915594849406));
#18810=DIRECTION('ref_axis',(-1.,0.,0.));
#18811=DIRECTION('',(-1.,0.,0.));
#18812=DIRECTION('',(0.,-0.997915594849406,-0.0645326704573514));
#18813=DIRECTION('center_axis',(0.,0.897258209424887,-0.441506178461464));
#18814=DIRECTION('ref_axis',(0.,0.441506178461464,0.897258209424887));
#18815=DIRECTION('',(0.,-0.441506178461464,-0.897258209424887));
#18816=DIRECTION('',(1.,0.,0.));
#18817=DIRECTION('center_axis',(0.,0.441506178461463,-0.897258209424887));
#18818=DIRECTION('ref_axis',(-1.,0.,0.));
#18819=DIRECTION('',(-1.,0.,0.));
#18820=DIRECTION('',(0.,-0.897258209424887,-0.441506178461463));
#18821=DIRECTION('center_axis',(0.,0.751264373058291,-0.660001395281353));
#18822=DIRECTION('ref_axis',(-1.,0.,0.));
#18823=DIRECTION('',(-1.,0.,0.));
#18824=DIRECTION('',(0.,-0.660001395281353,-0.751264373058291));
#18825=DIRECTION('center_axis',(0.,0.997915594849406,-0.0645326704573515));
#18826=DIRECTION('ref_axis',(0.,0.0645326704573514,0.997915594849406));
#18827=DIRECTION('',(0.,-0.0645326704573514,-0.997915594849406));
#18828=DIRECTION('',(1.,0.,0.));
#18829=DIRECTION('center_axis',(1.,0.,0.));
#18830=DIRECTION('ref_axis',(0.,-0.38268343236509,-0.923879532511287));
#18831=DIRECTION('center_axis',(1.,0.,0.));
#18832=DIRECTION('ref_axis',(0.,-0.38268343236509,-0.923879532511287));
#18833=DIRECTION('center_axis',(-1.,0.,0.));
#18834=DIRECTION('ref_axis',(0.,1.,0.));
#18835=DIRECTION('',(-0.707106781186548,-0.707106781186547,-8.65956056235493E-17));
#18836=DIRECTION('center_axis',(-1.,0.,0.));
#18837=DIRECTION('ref_axis',(0.,1.,0.));
#18838=DIRECTION('center_axis',(1.,0.,0.));
#18839=DIRECTION('ref_axis',(0.,0.,-1.));
#18840=DIRECTION('',(0.,4.06259722475401E-16,1.));
#18841=DIRECTION('',(0.,0.866025403784439,0.5));
#18842=DIRECTION('',(0.,0.866025403784439,-0.5));
#18843=DIRECTION('',(0.,1.354199074918E-16,-1.));
#18844=DIRECTION('',(0.,-0.866025403784439,-0.5));
#18845=DIRECTION('',(0.,-0.866025403784439,0.5));
#18846=DIRECTION('center_axis',(-0.707106781186548,0.353553390593274,-0.612372435695794));
#18847=DIRECTION('ref_axis',(-0.654653670707977,0.,0.755928946018455));
#18848=DIRECTION('',(0.,0.866025403784439,0.5));
#18849=DIRECTION('',(0.654653670707977,2.78478589689825E-15,-0.755928946018455));
#18850=DIRECTION('',(0.,-0.866025403784439,-0.5));
#18851=DIRECTION('',(0.654653670707977,0.654653670707979,-0.377964473009225));
#18852=DIRECTION('center_axis',(-0.707106781186547,-0.353553390593274,-0.612372435695795));
#18853=DIRECTION('ref_axis',(-0.654653670707977,0.,0.755928946018454));
#18854=DIRECTION('',(0.,0.866025403784439,-0.5));
#18855=DIRECTION('',(0.654653670707977,-0.654653670707978,-0.377964473009226));
#18856=DIRECTION('',(0.,-0.866025403784439,0.5));
#18857=DIRECTION('center_axis',(-0.707106781186547,-0.353553390593274,0.612372435695795));
#18858=DIRECTION('ref_axis',(0.654653670707978,0.,0.755928946018454));
#18859=DIRECTION('',(0.,-0.866025403784439,-0.5));
#18860=DIRECTION('',(0.654653670707976,5.13140401744201E-15,0.755928946018455));
#18861=DIRECTION('',(0.,0.866025403784439,0.5));
#18862=DIRECTION('',(-0.654653670707977,0.654653670707978,-0.377964473009226));
#18863=DIRECTION('center_axis',(-0.70710678118655,0.353553390593273,0.612372435695792));
#18864=DIRECTION('ref_axis',(0.654653670707975,0.,0.755928946018457));
#18865=DIRECTION('',(0.,0.866025403784439,-0.5));
#18866=DIRECTION('',(0.,-0.866025403784439,0.5));
#18867=DIRECTION('',(0.654653670707976,0.654653670707978,0.377964473009228));
#18868=DIRECTION('center_axis',(-0.707106781186548,-0.707106781186547,2.87269004685321E-16));
#18869=DIRECTION('ref_axis',(4.062597224754E-16,0.,1.));
#18870=DIRECTION('',(0.,-4.06259722475401E-16,-1.));
#18871=DIRECTION('',(0.,4.06259722475401E-16,1.));
#18872=DIRECTION('center_axis',(-0.707106781186548,0.707106781186547,9.57563348951068E-17));
#18873=DIRECTION('ref_axis',(1.354199074918E-16,0.,1.));
#18874=DIRECTION('',(0.,1.354199074918E-16,-1.));
#18875=DIRECTION('',(0.,-1.354199074918E-16,1.));
#18876=DIRECTION('center_axis',(0.,0.5,0.866025403784439));
#18877=DIRECTION('ref_axis',(0.,-0.866025403784439,0.5));
#18878=DIRECTION('',(1.,0.,0.));
#18879=DIRECTION('',(1.,0.,0.));
#18880=DIRECTION('center_axis',(0.,1.,-4.06259722475401E-16));
#18881=DIRECTION('ref_axis',(0.,4.06259722475401E-16,1.));
#18882=DIRECTION('',(1.,0.,0.));
#18883=DIRECTION('center_axis',(0.,0.5,-0.866025403784439));
#18884=DIRECTION('ref_axis',(0.,0.866025403784439,0.5));
#18885=DIRECTION('',(1.,0.,0.));
#18886=DIRECTION('center_axis',(-1.,0.,0.));
#18887=DIRECTION('ref_axis',(0.,0.,1.));
#18888=DIRECTION('center_axis',(1.,0.,0.));
#18889=DIRECTION('ref_axis',(0.,0.,-1.));
#18890=DIRECTION('center_axis',(0.,-0.5,-0.866025403784439));
#18891=DIRECTION('ref_axis',(0.,0.866025403784439,-0.5));
#18892=DIRECTION('',(1.,0.,0.));
#18893=DIRECTION('center_axis',(0.,-1.,-1.354199074918E-16));
#18894=DIRECTION('ref_axis',(0.,1.354199074918E-16,-1.));
#18895=DIRECTION('',(1.,0.,0.));
#18896=DIRECTION('center_axis',(0.,-0.5,0.866025403784439));
#18897=DIRECTION('ref_axis',(0.,-0.866025403784439,-0.5));
#18898=DIRECTION('center_axis',(1.,0.,0.));
#18899=DIRECTION('ref_axis',(0.,-0.38268343236509,-0.923879532511286));
#18900=DIRECTION('center_axis',(1.,0.,0.));
#18901=DIRECTION('ref_axis',(0.,-0.707106781186548,-0.707106781186547));
#18902=DIRECTION('center_axis',(1.,0.,0.));
#18903=DIRECTION('ref_axis',(0.,-0.707106781186548,-0.707106781186547));
#18904=DIRECTION('center_axis',(1.,0.,0.));
#18905=DIRECTION('ref_axis',(0.,-0.707106781186548,-0.707106781186547));
#18906=DIRECTION('center_axis',(1.,0.,0.));
#18907=DIRECTION('ref_axis',(0.,-0.923879532511287,-0.38268343236509));
#18908=DIRECTION('center_axis',(1.,0.,0.));
#18909=DIRECTION('ref_axis',(0.,-0.923879532511287,-0.38268343236509));
#18910=DIRECTION('center_axis',(1.,0.,0.));
#18911=DIRECTION('ref_axis',(0.,-0.923879532511287,-0.38268343236509));
#18912=DIRECTION('center_axis',(1.,0.,0.));
#18913=DIRECTION('ref_axis',(0.,-1.,1.83697019872103E-16));
#18914=DIRECTION('center_axis',(1.,0.,0.));
#18915=DIRECTION('ref_axis',(0.,-1.,1.83697019872103E-16));
#18916=DIRECTION('center_axis',(1.,0.,0.));
#18917=DIRECTION('ref_axis',(0.,-1.,1.83697019872103E-16));
#18918=DIRECTION('center_axis',(1.,0.,0.));
#18919=DIRECTION('ref_axis',(0.,-0.923879532511286,0.38268343236509));
#18920=DIRECTION('center_axis',(1.,0.,0.));
#18921=DIRECTION('ref_axis',(0.,-0.923879532511287,0.38268343236509));
#18922=DIRECTION('center_axis',(1.,0.,0.));
#18923=DIRECTION('ref_axis',(0.,-0.923879532511287,0.38268343236509));
#18924=DIRECTION('center_axis',(1.,0.,0.));
#18925=DIRECTION('ref_axis',(0.,-0.707106781186547,0.707106781186548));
#18926=DIRECTION('center_axis',(1.,0.,0.));
#18927=DIRECTION('ref_axis',(0.,-0.707106781186547,0.707106781186548));
#18928=DIRECTION('center_axis',(1.,0.,0.));
#18929=DIRECTION('ref_axis',(0.,-0.707106781186547,0.707106781186548));
#18930=DIRECTION('center_axis',(1.,0.,0.));
#18931=DIRECTION('ref_axis',(0.,-0.38268343236509,0.923879532511287));
#18932=DIRECTION('center_axis',(1.,0.,0.));
#18933=DIRECTION('ref_axis',(0.,-0.38268343236509,0.923879532511287));
#18934=DIRECTION('center_axis',(1.,0.,0.));
#18935=DIRECTION('ref_axis',(0.,-0.38268343236509,0.923879532511287));
#18936=DIRECTION('center_axis',(1.,0.,0.));
#18937=DIRECTION('ref_axis',(0.,1.22464679914735E-16,1.));
#18938=DIRECTION('center_axis',(1.,0.,0.));
#18939=DIRECTION('ref_axis',(0.,1.22464679914735E-16,1.));
#18940=DIRECTION('center_axis',(1.,0.,0.));
#18941=DIRECTION('ref_axis',(0.,1.22464679914735E-16,1.));
#18942=DIRECTION('center_axis',(1.,0.,0.));
#18943=DIRECTION('ref_axis',(0.,0.38268343236509,0.923879532511287));
#18944=DIRECTION('center_axis',(1.,0.,0.));
#18945=DIRECTION('ref_axis',(0.,0.38268343236509,0.923879532511287));
#18946=DIRECTION('center_axis',(1.,0.,0.));
#18947=DIRECTION('ref_axis',(0.,0.38268343236509,0.923879532511287));
#18948=DIRECTION('center_axis',(1.,0.,0.));
#18949=DIRECTION('ref_axis',(0.,0.707106781186548,0.707106781186547));
#18950=DIRECTION('center_axis',(1.,0.,0.));
#18951=DIRECTION('ref_axis',(0.,0.707106781186548,0.707106781186547));
#18952=DIRECTION('center_axis',(1.,0.,0.));
#18953=DIRECTION('ref_axis',(0.,0.707106781186548,0.707106781186547));
#18954=DIRECTION('center_axis',(1.,0.,0.));
#18955=DIRECTION('ref_axis',(0.,0.923879532511287,0.38268343236509));
#18956=DIRECTION('center_axis',(1.,0.,0.));
#18957=DIRECTION('ref_axis',(0.,0.923879532511287,0.38268343236509));
#18958=DIRECTION('center_axis',(1.,0.,0.));
#18959=DIRECTION('ref_axis',(0.,0.923879532511287,0.38268343236509));
#18960=DIRECTION('center_axis',(1.,0.,0.));
#18961=DIRECTION('ref_axis',(0.,1.,-6.12323399573677E-17));
#18962=DIRECTION('center_axis',(1.,0.,0.));
#18963=DIRECTION('ref_axis',(0.,1.,-6.12323399573677E-17));
#18964=DIRECTION('center_axis',(1.,0.,0.));
#18965=DIRECTION('ref_axis',(0.,1.,-6.12323399573677E-17));
#18966=DIRECTION('center_axis',(1.,0.,0.));
#18967=DIRECTION('ref_axis',(0.,0.923879532511287,-0.38268343236509));
#18968=DIRECTION('center_axis',(1.,0.,0.));
#18969=DIRECTION('ref_axis',(0.,0.923879532511287,-0.38268343236509));
#18970=DIRECTION('center_axis',(1.,0.,0.));
#18971=DIRECTION('ref_axis',(0.,0.923879532511287,-0.38268343236509));
#18972=DIRECTION('center_axis',(1.,0.,0.));
#18973=DIRECTION('ref_axis',(0.,0.707106781186548,-0.707106781186548));
#18974=DIRECTION('center_axis',(1.,0.,0.));
#18975=DIRECTION('ref_axis',(0.,0.707106781186548,-0.707106781186548));
#18976=DIRECTION('center_axis',(1.,0.,0.));
#18977=DIRECTION('ref_axis',(0.,0.707106781186548,-0.707106781186548));
#18978=DIRECTION('center_axis',(1.,0.,0.));
#18979=DIRECTION('ref_axis',(0.,0.38268343236509,-0.923879532511287));
#18980=DIRECTION('center_axis',(1.,0.,0.));
#18981=DIRECTION('ref_axis',(0.,0.38268343236509,-0.923879532511287));
#18982=DIRECTION('center_axis',(1.,0.,0.));
#18983=DIRECTION('ref_axis',(0.,0.38268343236509,-0.923879532511287));
#18984=DIRECTION('center_axis',(1.,0.,0.));
#18985=DIRECTION('ref_axis',(0.,0.,-1.));
#18986=DIRECTION('center_axis',(1.,0.,0.));
#18987=DIRECTION('ref_axis',(0.,0.,-1.));
#18988=DIRECTION('center_axis',(1.,0.,0.));
#18989=DIRECTION('ref_axis',(0.,0.,-1.));
#18990=DIRECTION('center_axis',(1.,0.,0.));
#18991=DIRECTION('ref_axis',(0.,1.,0.));
#18992=DIRECTION('',(-0.707106781186547,0.707106781186548,8.65956056235494E-17));
#26207=CARTESIAN_POINT('',(0.,0.,0.));
#26208=CARTESIAN_POINT('Origin',(7.84,0.,0.));
#26209=CARTESIAN_POINT('',(7.68,2.15,-2.63299061816681E-16));
#26210=CARTESIAN_POINT('',(7.68,-2.15,-2.63299061816681E-16));
#26211=CARTESIAN_POINT('Origin',(7.68,0.,0.));
#26212=CARTESIAN_POINT('Origin',(7.68,0.,0.));
#26213=CARTESIAN_POINT('',(8.,2.47,3.02487759389396E-16));
#26214=CARTESIAN_POINT('',(7.84,2.31,-2.82893410603039E-16));
#26215=CARTESIAN_POINT('Origin',(8.,0.,0.));
#26216=CARTESIAN_POINT('Origin',(4.,0.,0.));
#26217=CARTESIAN_POINT('',(3.32,-2.15,-2.63299061816681E-16));
#26218=CARTESIAN_POINT('',(4.,-2.15,-2.63299061816681E-16));
#26219=CARTESIAN_POINT('Origin',(3.32,0.,0.));
#26220=CARTESIAN_POINT('Origin',(8.,2.15,0.));
#26221=CARTESIAN_POINT('',(8.,-5.9,-7.22541611496939E-16));
#26222=CARTESIAN_POINT('Origin',(8.,0.,0.));
#26223=CARTESIAN_POINT('Origin',(3.95,6.34315468735702,-0.634180373472705));
#26224=CARTESIAN_POINT('',(7.6395955992633,6.25001191701594,-0.360574957917378));
#26225=CARTESIAN_POINT('',(7.4,6.43629745752619,-0.907785788741997));
#26226=CARTESIAN_POINT('Ctrl Pts',(7.6395955992633,6.25001191701594,-0.360574957917378));
#26227=CARTESIAN_POINT('Ctrl Pts',(7.53289072318166,6.34140579300765,-0.629043024168655));
#26228=CARTESIAN_POINT('Ctrl Pts',(7.4,6.43629745752619,-0.907785788741997));
#26229=CARTESIAN_POINT('',(0.6,6.43629745752619,-0.907785788741997));
#26230=CARTESIAN_POINT('',(3.95,6.43629745752619,-0.907785788741997));
#26231=CARTESIAN_POINT('',(0.6,6.25001191718784,-0.360574958203413));
#26232=CARTESIAN_POINT('',(0.6,6.2727384556044,-0.427333805613703));
#26233=CARTESIAN_POINT('',(3.95,6.25001191718784,-0.360574958203413));
#26234=CARTESIAN_POINT('Origin',(3.95,0.,0.));
#26235=CARTESIAN_POINT('',(0.6,6.43629745752619,0.907785788741997));
#26236=CARTESIAN_POINT('Origin',(0.6,0.,0.));
#26237=CARTESIAN_POINT('',(7.4,6.29734418894816,-1.61042111446691));
#26238=CARTESIAN_POINT('Origin',(7.4,0.,0.));
#26239=CARTESIAN_POINT('',(7.38278617788904,6.29375806765092,-1.62437969264548));
#26240=CARTESIAN_POINT('Ctrl Pts',(7.38278617788871,6.29375806765085,-1.62437969264574));
#26241=CARTESIAN_POINT('Ctrl Pts',(7.38853745459905,6.29495796151265,-1.61972967166525));
#26242=CARTESIAN_POINT('Ctrl Pts',(7.39427239342974,6.29615711204027,-1.61507445283177));
#26243=CARTESIAN_POINT('Ctrl Pts',(7.3999909815365,6.2973543093563,-1.61041566515606));
#26244=CARTESIAN_POINT('',(0.6,6.29375806765092,-1.62437969264548));
#26245=CARTESIAN_POINT('',(3.95,6.29375806765092,-1.62437969264548));
#26246=CARTESIAN_POINT('',(0.6,5.59896890467484,-3.30174911289217));
#26247=CARTESIAN_POINT('Origin',(0.6,0.,0.));
#26248=CARTESIAN_POINT('',(7.38278617788903,5.59896890467484,-3.30174911289217));
#26249=CARTESIAN_POINT('',(3.95,5.59896890467484,-3.30174911289217));
#26250=CARTESIAN_POINT('',(7.40000076486337,5.5916352232277,-3.31415213071781));
#26251=CARTESIAN_POINT('Ctrl Pts',(7.40000076486337,5.5916352232277,-3.31415213071781));
#26252=CARTESIAN_POINT('Ctrl Pts',(7.39427320375822,5.59408570519366,-3.31001880145165));
#26253=CARTESIAN_POINT('Ctrl Pts',(7.38853488546801,5.59653040730634,-3.3058839072742));
#26254=CARTESIAN_POINT('Ctrl Pts',(7.38278617788892,5.59896890467488,-3.30174911289203));
#26255=CARTESIAN_POINT('',(7.4,5.19305106503475,-3.90924809086626));
#26256=CARTESIAN_POINT('Origin',(7.4,0.,0.));
#26257=CARTESIAN_POINT('',(0.6,5.19305106503475,-3.90924809086626));
#26258=CARTESIAN_POINT('',(3.95,5.19305106503475,-3.90924809086626));
#26259=CARTESIAN_POINT('',(0.6,3.90924809086626,-5.19305106503475));
#26260=CARTESIAN_POINT('Origin',(0.6,0.,0.));
#26261=CARTESIAN_POINT('',(7.4,3.90924809086626,-5.19305106503475));
#26262=CARTESIAN_POINT('',(3.95,3.90924809086626,-5.19305106503475));
#26263=CARTESIAN_POINT('',(7.4,3.30174911289217,-5.59896890467484));
#26264=CARTESIAN_POINT('Origin',(7.4,0.,0.));
#26265=CARTESIAN_POINT('',(0.6,3.30174911289217,-5.59896890467484));
#26266=CARTESIAN_POINT('',(3.95,3.30174911289217,-5.59896890467484));
#26267=CARTESIAN_POINT('',(0.6,1.62437969264548,-6.29375806765092));
#26268=CARTESIAN_POINT('Origin',(0.6,0.,0.));
#26269=CARTESIAN_POINT('',(7.4,1.62437969264548,-6.29375806765092));
#26270=CARTESIAN_POINT('',(3.95,1.62437969264548,-6.29375806765092));
#26271=CARTESIAN_POINT('',(7.4,0.907785788741996,-6.43629745752619));
#26272=CARTESIAN_POINT('Origin',(7.4,0.,0.));
#26273=CARTESIAN_POINT('',(0.6,0.907785788741996,-6.43629745752619));
#26274=CARTESIAN_POINT('',(3.95,0.907785788741996,-6.43629745752619));
#26275=CARTESIAN_POINT('',(0.6,-0.907785788741998,-6.43629745752619));
#26276=CARTESIAN_POINT('Origin',(0.6,0.,0.));
#26277=CARTESIAN_POINT('',(7.4,-0.907785788741998,-6.43629745752619));
#26278=CARTESIAN_POINT('',(3.95,-0.907785788741998,-6.43629745752619));
#26279=CARTESIAN_POINT('',(7.4,-1.62437969264548,-6.29375806765091));
#26280=CARTESIAN_POINT('Origin',(7.4,0.,0.));
#26281=CARTESIAN_POINT('',(0.6,-1.62437969264548,-6.29375806765092));
#26282=CARTESIAN_POINT('',(3.95,-1.62437969264548,-6.29375806765092));
#26283=CARTESIAN_POINT('',(0.6,-3.30174911289217,-5.59896890467484));
#26284=CARTESIAN_POINT('Origin',(0.6,0.,0.));
#26285=CARTESIAN_POINT('',(7.4,-3.30174911289217,-5.59896890467484));
#26286=CARTESIAN_POINT('',(3.95,-3.30174911289217,-5.59896890467484));
#26287=CARTESIAN_POINT('',(7.4,-3.90924809086626,-5.19305106503474));
#26288=CARTESIAN_POINT('Origin',(7.4,0.,0.));
#26289=CARTESIAN_POINT('',(0.6,-3.90924809086626,-5.19305106503474));
#26290=CARTESIAN_POINT('',(3.95,-3.90924809086626,-5.19305106503474));
#26291=CARTESIAN_POINT('',(0.6,-5.19305106503474,-3.90924809086626));
#26292=CARTESIAN_POINT('Origin',(0.6,0.,0.));
#26293=CARTESIAN_POINT('',(7.4,-5.19305106503474,-3.90924809086626));
#26294=CARTESIAN_POINT('',(3.95,-5.19305106503474,-3.90924809086626));
#26295=CARTESIAN_POINT('',(7.4,-5.59896890467484,-3.30174911289217));
#26296=CARTESIAN_POINT('Origin',(7.4,0.,0.));
#26297=CARTESIAN_POINT('',(0.6,-5.59896890467484,-3.30174911289217));
#26298=CARTESIAN_POINT('',(3.95,-5.59896890467484,-3.30174911289217));
#26299=CARTESIAN_POINT('',(0.6,-6.29375806765092,-1.62437969264548));
#26300=CARTESIAN_POINT('Origin',(0.6,0.,0.));
#26301=CARTESIAN_POINT('',(7.4,-6.29375806765092,-1.62437969264547));
#26302=CARTESIAN_POINT('',(3.95,-6.29375806765092,-1.62437969264548));
#26303=CARTESIAN_POINT('',(7.4,-6.43629745752619,-0.907785788741997));
#26304=CARTESIAN_POINT('Origin',(7.4,0.,0.));
#26305=CARTESIAN_POINT('',(0.6,-6.43629745752619,-0.907785788741997));
#26306=CARTESIAN_POINT('',(3.95,-6.43629745752619,-0.907785788741997));
#26307=CARTESIAN_POINT('',(0.6,-6.5,-7.9602041944578E-16));
#26308=CARTESIAN_POINT('Origin',(0.6,0.,0.));
#26309=CARTESIAN_POINT('',(0.500000000000001,-6.5,-7.9602041944578E-16));
#26310=CARTESIAN_POINT('',(3.95,-6.5,-7.9602041944578E-16));
#26311=CARTESIAN_POINT('Origin',(0.5,0.,0.));
#26312=CARTESIAN_POINT('',(0.6,-6.43629745752619,0.907785788741998));
#26313=CARTESIAN_POINT('Origin',(0.6,0.,0.));
#26314=CARTESIAN_POINT('',(7.4,-6.43629745752619,0.907785788741998));
#26315=CARTESIAN_POINT('',(3.95,-6.43629745752619,0.907785788741998));
#26316=CARTESIAN_POINT('',(7.4,-6.29375806765092,1.62437969264548));
#26317=CARTESIAN_POINT('Origin',(7.4,0.,0.));
#26318=CARTESIAN_POINT('',(0.6,-6.29375806765092,1.62437969264548));
#26319=CARTESIAN_POINT('',(3.95,-6.29375806765092,1.62437969264548));
#26320=CARTESIAN_POINT('',(0.6,-5.59896890467484,3.30174911289217));
#26321=CARTESIAN_POINT('Origin',(0.6,0.,0.));
#26322=CARTESIAN_POINT('',(7.4,-5.59896890467484,3.30174911289217));
#26323=CARTESIAN_POINT('',(3.95,-5.59896890467484,3.30174911289217));
#26324=CARTESIAN_POINT('',(7.4,-5.19305106503475,3.90924809086626));
#26325=CARTESIAN_POINT('Origin',(7.4,0.,0.));
#26326=CARTESIAN_POINT('',(0.6,-5.19305106503475,3.90924809086626));
#26327=CARTESIAN_POINT('',(3.95,-5.19305106503475,3.90924809086626));
#26328=CARTESIAN_POINT('',(0.6,-3.90924809086626,5.19305106503475));
#26329=CARTESIAN_POINT('Origin',(0.6,0.,0.));
#26330=CARTESIAN_POINT('',(7.4,-3.90924809086626,5.19305106503475));
#26331=CARTESIAN_POINT('',(3.95,-3.90924809086626,5.19305106503475));
#26332=CARTESIAN_POINT('',(7.4,-3.30174911289217,5.59896890467484));
#26333=CARTESIAN_POINT('Origin',(7.4,0.,0.));
#26334=CARTESIAN_POINT('',(0.6,-3.30174911289217,5.59896890467484));
#26335=CARTESIAN_POINT('',(3.95,-3.30174911289217,5.59896890467484));
#26336=CARTESIAN_POINT('',(0.6,-1.62437969264548,6.29375806765092));
#26337=CARTESIAN_POINT('Origin',(0.6,0.,0.));
#26338=CARTESIAN_POINT('',(7.4,-1.62437969264548,6.29375806765092));
#26339=CARTESIAN_POINT('',(3.95,-1.62437969264548,6.29375806765092));
#26340=CARTESIAN_POINT('',(7.4,-0.907785788741997,6.43629745752619));
#26341=CARTESIAN_POINT('Origin',(7.4,0.,0.));
#26342=CARTESIAN_POINT('',(0.6,-0.907785788741997,6.43629745752619));
#26343=CARTESIAN_POINT('',(3.95,-0.907785788741997,6.43629745752619));
#26344=CARTESIAN_POINT('',(0.6,0.907785788741998,6.43629745752619));
#26345=CARTESIAN_POINT('Origin',(0.6,0.,0.));
#26346=CARTESIAN_POINT('',(7.4,0.907785788741998,6.43629745752619));
#26347=CARTESIAN_POINT('',(3.95,0.907785788741998,6.43629745752619));
#26348=CARTESIAN_POINT('',(7.4,1.62437969264548,6.29375806765092));
#26349=CARTESIAN_POINT('Origin',(7.4,0.,0.));
#26350=CARTESIAN_POINT('',(0.6,1.62437969264548,6.29375806765092));
#26351=CARTESIAN_POINT('',(3.95,1.62437969264548,6.29375806765092));
#26352=CARTESIAN_POINT('',(0.6,3.30174911289217,5.59896890467484));
#26353=CARTESIAN_POINT('Origin',(0.6,0.,0.));
#26354=CARTESIAN_POINT('',(7.4,3.30174911289217,5.59896890467484));
#26355=CARTESIAN_POINT('',(3.95,3.30174911289217,5.59896890467484));
#26356=CARTESIAN_POINT('',(7.4,3.90924809086626,5.19305106503475));
#26357=CARTESIAN_POINT('Origin',(7.4,0.,0.));
#26358=CARTESIAN_POINT('',(0.6,3.90924809086626,5.19305106503475));
#26359=CARTESIAN_POINT('',(3.95,3.90924809086626,5.19305106503475));
#26360=CARTESIAN_POINT('',(0.6,5.19305106503475,3.90924809086626));
#26361=CARTESIAN_POINT('Origin',(0.6,0.,0.));
#26362=CARTESIAN_POINT('',(7.4,5.19305106503475,3.90924809086626));
#26363=CARTESIAN_POINT('',(3.95,5.19305106503475,3.90924809086626));
#26364=CARTESIAN_POINT('',(7.4,5.59896890467484,3.30174911289217));
#26365=CARTESIAN_POINT('Origin',(7.4,0.,0.));
#26366=CARTESIAN_POINT('',(0.6,5.59896890467484,3.30174911289217));
#26367=CARTESIAN_POINT('',(3.95,5.59896890467484,3.30174911289217));
#26368=CARTESIAN_POINT('',(0.6,6.29375806765092,1.62437969264548));
#26369=CARTESIAN_POINT('Origin',(0.6,0.,0.));
#26370=CARTESIAN_POINT('',(7.4,6.29375806765092,1.62437969264548));
#26371=CARTESIAN_POINT('',(3.95,6.29375806765092,1.62437969264548));
#26372=CARTESIAN_POINT('',(7.4,6.43629745752619,0.907785788741997));
#26373=CARTESIAN_POINT('Origin',(7.4,0.,0.));
#26374=CARTESIAN_POINT('',(3.95,6.43629745752619,0.907785788741997));
#26375=CARTESIAN_POINT('Origin',(7.7,0.,0.));
#26376=CARTESIAN_POINT('',(7.75,-6.15,8.74596390859847E-17));
#26377=CARTESIAN_POINT('',(7.7,-6.2,-7.59281015471359E-16));
#26378=CARTESIAN_POINT('',(7.6395955992633,-6.25001191701594,-0.360574957917378));
#26379=CARTESIAN_POINT('Ctrl Pts',(7.75,-6.15,9.28077059647592E-16));
#26380=CARTESIAN_POINT('Ctrl Pts',(7.75,-6.15,-0.080715219171627));
#26381=CARTESIAN_POINT('Ctrl Pts',(7.73340207567264,-6.16485627699069,-0.16401583254945));
#26382=CARTESIAN_POINT('Ctrl Pts',(7.6858526263557,-6.20786999945922,-0.282558774022249));
#26383=CARTESIAN_POINT('Ctrl Pts',(7.66390188127962,-6.22779773364639,-0.323611089501759));
#26384=CARTESIAN_POINT('Ctrl Pts',(7.63959559912056,-6.2500119169745,-0.360574957848419));
#26385=CARTESIAN_POINT('Ctrl Pts',(7.4,-6.43629745752619,-0.907785788741997));
#26386=CARTESIAN_POINT('Ctrl Pts',(7.53289072319445,-6.34140579300535,-0.629043024174526));
#26387=CARTESIAN_POINT('Ctrl Pts',(7.6395955992633,-6.25001191701594,-0.360574957917378));
#26388=CARTESIAN_POINT('',(7.6395955992633,-5.91224415060338,-2.05864818917039));
#26389=CARTESIAN_POINT('Ctrl Pts',(7.6395955992633,-5.91224415060338,-2.05864818917039));
#26390=CARTESIAN_POINT('Ctrl Pts',(7.53289072318166,-6.09941936310245,-1.84559095978961));
#26391=CARTESIAN_POINT('Ctrl Pts',(7.4,-6.29375806765092,-1.62437969264548));
#26392=CARTESIAN_POINT('',(7.6395955992633,-5.63627202556194,-2.72490383628236));
#26393=CARTESIAN_POINT('Ctrl Pts',(7.63959559912056,-5.91224415053871,-2.05864818921824));
#26394=CARTESIAN_POINT('Ctrl Pts',(7.66390188127962,-5.87757546121802,-2.08429735070297));
#26395=CARTESIAN_POINT('Ctrl Pts',(7.6858526263557,-5.84345459447894,-2.11459873101868));
#26396=CARTESIAN_POINT('Ctrl Pts',(7.73340207567264,-5.75835067694767,-2.20765748941603));
#26397=CARTESIAN_POINT('Ctrl Pts',(7.75,-5.71274750206111,-2.27893197009047));
#26398=CARTESIAN_POINT('Ctrl Pts',(7.75,-5.65097074782772,-2.42807424800013));
#26399=CARTESIAN_POINT('Ctrl Pts',(7.73340207567264,-5.63281839342319,-2.5107192308165));
#26400=CARTESIAN_POINT('Ctrl Pts',(7.68585262635569,-5.62719347150353,-2.63669926711996));
#26401=CARTESIAN_POINT('Ctrl Pts',(7.66390188127962,-5.62989425625414,-2.68225267487168));
#26402=CARTESIAN_POINT('Ctrl Pts',(7.63959559912056,-5.63627202555004,-2.72490383620279));
#26403=CARTESIAN_POINT('Ctrl Pts',(7.4,-5.59896890467484,-3.30174911289217));
#26404=CARTESIAN_POINT('Ctrl Pts',(7.53289072319445,-5.61797067590973,-3.00791090999099));
#26405=CARTESIAN_POINT('Ctrl Pts',(7.6395955992633,-5.63627202556194,-2.72490383628236));
#26406=CARTESIAN_POINT('',(7.6395955992633,-4.67439080688814,-4.16446081114928));
#26407=CARTESIAN_POINT('Ctrl Pts',(7.6395955992633,-4.67439080688814,-4.16446081114928));
#26408=CARTESIAN_POINT('Ctrl Pts',(7.53289072318166,-4.92885162653911,-4.03925045044361));
#26409=CARTESIAN_POINT('Ctrl Pts',(7.4,-5.19305106503474,-3.90924809086626));
#26410=CARTESIAN_POINT('',(7.6395955992633,-4.16446081114928,-4.67439080688814));
#26411=CARTESIAN_POINT('Ctrl Pts',(7.63959559912056,-4.67439080681007,-4.16446081116873));
#26412=CARTESIAN_POINT('Ctrl Pts',(7.66390188127962,-4.63254560517343,-4.17489041346571));
#26413=CARTESIAN_POINT('Ctrl Pts',(7.6858526263557,-4.58942619853704,-4.18982774814726));
#26414=CARTESIAN_POINT('Ctrl Pts',(7.73340207567264,-4.47518838591824,-4.2432349710829));
#26415=CARTESIAN_POINT('Ctrl Pts',(7.75,-4.40578098311848,-4.29163242547605));
#26416=CARTESIAN_POINT('Ctrl Pts',(7.75,-4.29163242547605,-4.40578098311848));
#26417=CARTESIAN_POINT('Ctrl Pts',(7.73340207567264,-4.2432349710829,-4.47518838591824));
#26418=CARTESIAN_POINT('Ctrl Pts',(7.68585262635569,-4.18982774814726,-4.58942619853704));
#26419=CARTESIAN_POINT('Ctrl Pts',(7.66390188127962,-4.17489041346571,-4.63254560517343));
#26420=CARTESIAN_POINT('Ctrl Pts',(7.63959559912056,-4.16446081116873,-4.67439080681007));
#26421=CARTESIAN_POINT('Ctrl Pts',(7.4,-3.90924809086626,-5.19305106503474));
#26422=CARTESIAN_POINT('Ctrl Pts',(7.53289072319445,-4.03925045043784,-4.92885162654163));
#26423=CARTESIAN_POINT('Ctrl Pts',(7.6395955992633,-4.16446081114928,-4.67439080688814));
#26424=CARTESIAN_POINT('',(7.6395955992633,-2.72490383628237,-5.63627202556194));
#26425=CARTESIAN_POINT('Ctrl Pts',(7.6395955992633,-2.72490383628237,-5.63627202556194));
#26426=CARTESIAN_POINT('Ctrl Pts',(7.53289072318165,-3.00791090998646,-5.61797067591409));
#26427=CARTESIAN_POINT('Ctrl Pts',(7.4,-3.30174911289217,-5.59896890467484));
#26428=CARTESIAN_POINT('',(7.6395955992633,-2.0586481891704,-5.91224415060338));
#26429=CARTESIAN_POINT('Ctrl Pts',(7.63959559912056,-2.7249038362028,-5.63627202555004));
#26430=CARTESIAN_POINT('Ctrl Pts',(7.66390188127961,-2.68225267487168,-5.62989425625414));
#26431=CARTESIAN_POINT('Ctrl Pts',(7.6858526263557,-2.63669926711997,-5.62719347150352));
#26432=CARTESIAN_POINT('Ctrl Pts',(7.73340207567264,-2.51071923081651,-5.63281839342319));
#26433=CARTESIAN_POINT('Ctrl Pts',(7.75,-2.42807424800014,-5.65097074782771));
#26434=CARTESIAN_POINT('Ctrl Pts',(7.75,-2.27893197009048,-5.71274750206111));
#26435=CARTESIAN_POINT('Ctrl Pts',(7.73340207567264,-2.20765748941603,-5.75835067694767));
#26436=CARTESIAN_POINT('Ctrl Pts',(7.6858526263557,-2.11459873101869,-5.84345459447893));
#26437=CARTESIAN_POINT('Ctrl Pts',(7.66390188127962,-2.08429735070298,-5.87757546121802));
#26438=CARTESIAN_POINT('Ctrl Pts',(7.63959559912056,-2.05864818921825,-5.91224415053871));
#26439=CARTESIAN_POINT('Ctrl Pts',(7.4,-1.62437969264548,-6.29375806765091));
#26440=CARTESIAN_POINT('Ctrl Pts',(7.53289072319445,-1.84559095978331,-6.09941936310257));
#26441=CARTESIAN_POINT('Ctrl Pts',(7.6395955992633,-2.0586481891704,-5.91224415060338));
#26442=CARTESIAN_POINT('',(7.6395955992633,-0.360574957917379,-6.25001191701594));
#26443=CARTESIAN_POINT('Ctrl Pts',(7.6395955992633,-0.360574957917379,-6.25001191701594));
#26444=CARTESIAN_POINT('Ctrl Pts',(7.53289072318166,-0.629043024168655,
-6.34140579300765));
#26445=CARTESIAN_POINT('Ctrl Pts',(7.4,-0.907785788741998,-6.43629745752619));
#26446=CARTESIAN_POINT('',(7.6395955992633,0.360574957917378,-6.25001191701594));
#26447=CARTESIAN_POINT('Ctrl Pts',(7.63959559912056,-0.360574957848421,
-6.2500119169745));
#26448=CARTESIAN_POINT('Ctrl Pts',(7.66390188127962,-0.323611089501761,
-6.22779773364639));
#26449=CARTESIAN_POINT('Ctrl Pts',(7.68585262635569,-0.282558774022252,
-6.20786999945922));
#26450=CARTESIAN_POINT('Ctrl Pts',(7.73340207567264,-0.164015832549453,
-6.16485627699069));
#26451=CARTESIAN_POINT('Ctrl Pts',(7.75,-0.0807152191716292,-6.15));
#26452=CARTESIAN_POINT('Ctrl Pts',(7.75,0.0807152191716266,-6.15));
#26453=CARTESIAN_POINT('Ctrl Pts',(7.73340207567264,0.16401583254945,-6.16485627699069));
#26454=CARTESIAN_POINT('Ctrl Pts',(7.6858526263557,0.28255877402225,-6.20786999945922));
#26455=CARTESIAN_POINT('Ctrl Pts',(7.66390188127962,0.32361108950176,-6.22779773364639));
#26456=CARTESIAN_POINT('Ctrl Pts',(7.63959559912056,0.36057495784842,-6.2500119169745));
#26457=CARTESIAN_POINT('Ctrl Pts',(7.4,0.907785788741996,-6.43629745752619));
#26458=CARTESIAN_POINT('Ctrl Pts',(7.53289072319445,0.629043024174527,-6.34140579300535));
#26459=CARTESIAN_POINT('Ctrl Pts',(7.6395955992633,0.360574957917378,-6.25001191701594));
#26460=CARTESIAN_POINT('',(7.6395955992633,2.05864818917039,-5.91224415060338));
#26461=CARTESIAN_POINT('Ctrl Pts',(7.6395955992633,2.05864818917039,-5.91224415060338));
#26462=CARTESIAN_POINT('Ctrl Pts',(7.53289072318166,1.84559095978961,-6.09941936310245));
#26463=CARTESIAN_POINT('Ctrl Pts',(7.4,1.62437969264548,-6.29375806765092));
#26464=CARTESIAN_POINT('',(7.6395955992633,2.72490383628236,-5.63627202556194));
#26465=CARTESIAN_POINT('Ctrl Pts',(7.63959559912056,2.05864818921824,-5.91224415053871));
#26466=CARTESIAN_POINT('Ctrl Pts',(7.66390188127961,2.08429735070297,-5.87757546121802));
#26467=CARTESIAN_POINT('Ctrl Pts',(7.6858526263557,2.11459873101869,-5.84345459447894));
#26468=CARTESIAN_POINT('Ctrl Pts',(7.73340207567264,2.20765748941603,-5.75835067694767));
#26469=CARTESIAN_POINT('Ctrl Pts',(7.75,2.27893197009047,-5.71274750206111));
#26470=CARTESIAN_POINT('Ctrl Pts',(7.75,2.42807424800013,-5.65097074782771));
#26471=CARTESIAN_POINT('Ctrl Pts',(7.73340207567264,2.5107192308165,-5.63281839342319));
#26472=CARTESIAN_POINT('Ctrl Pts',(7.68585262635569,2.63669926711996,-5.62719347150352));
#26473=CARTESIAN_POINT('Ctrl Pts',(7.66390188127962,2.68225267487168,-5.62989425625414));
#26474=CARTESIAN_POINT('Ctrl Pts',(7.63959559912056,2.72490383620279,-5.63627202555004));
#26475=CARTESIAN_POINT('Ctrl Pts',(7.4,3.30174911289217,-5.59896890467484));
#26476=CARTESIAN_POINT('Ctrl Pts',(7.53289072319445,3.007910909991,-5.61797067590972));
#26477=CARTESIAN_POINT('Ctrl Pts',(7.6395955992633,2.72490383628236,-5.63627202556194));
#26478=CARTESIAN_POINT('',(7.6395955992633,4.16446081114928,-4.67439080688814));
#26479=CARTESIAN_POINT('Ctrl Pts',(7.6395955992633,4.16446081114928,-4.67439080688814));
#26480=CARTESIAN_POINT('Ctrl Pts',(7.53289072318166,4.03925045044361,-4.92885162653911));
#26481=CARTESIAN_POINT('Ctrl Pts',(7.4,3.90924809086626,-5.19305106503475));
#26482=CARTESIAN_POINT('',(7.6395955992633,4.67439080688814,-4.16446081114928));
#26483=CARTESIAN_POINT('Ctrl Pts',(7.63959559912056,4.16446081116873,-4.67439080681008));
#26484=CARTESIAN_POINT('Ctrl Pts',(7.66390188127962,4.17489041346571,-4.63254560517344));
#26485=CARTESIAN_POINT('Ctrl Pts',(7.68585262635569,4.18982774814726,-4.58942619853704));
#26486=CARTESIAN_POINT('Ctrl Pts',(7.73340207567264,4.24323497108289,-4.47518838591825));
#26487=CARTESIAN_POINT('Ctrl Pts',(7.75,4.29163242547605,-4.40578098311848));
#26488=CARTESIAN_POINT('Ctrl Pts',(7.75,4.40578098311848,-4.29163242547605));
#26489=CARTESIAN_POINT('Ctrl Pts',(7.73340207567264,4.47518838591824,-4.2432349710829));
#26490=CARTESIAN_POINT('Ctrl Pts',(7.6858526263557,4.58942619853704,-4.18982774814726));
#26491=CARTESIAN_POINT('Ctrl Pts',(7.66390188127962,4.63254560517343,-4.17489041346571));
#26492=CARTESIAN_POINT('Ctrl Pts',(7.63959559912056,4.67439080681008,-4.16446081116873));
#26493=CARTESIAN_POINT('Ctrl Pts',(7.4,5.19305106503475,-3.90924809086626));
#26494=CARTESIAN_POINT('Ctrl Pts',(7.53289072319445,4.92885162654163,-4.03925045043784));
#26495=CARTESIAN_POINT('Ctrl Pts',(7.6395955992633,4.67439080688814,-4.16446081114928));
#26496=CARTESIAN_POINT('Ctrl Pts',(7.40000051046853,6.29734425077455,-1.6104165295937));
#26497=CARTESIAN_POINT('Ctrl Pts',(7.47330660022597,6.21996344948776,-1.6170670263044));
#26498=CARTESIAN_POINT('Ctrl Pts',(7.6818261033525,5.99172758842293,-1.66250658304213));
#26499=CARTESIAN_POINT('Ctrl Pts',(7.97308777074854,5.61920950447284,-1.91938073772091));
#26500=CARTESIAN_POINT('Ctrl Pts',(7.98425119443302,5.38246983194813,-2.46771855869631));
#26501=CARTESIAN_POINT('Ctrl Pts',(7.81463329279646,5.37650527564507,-2.85267802239966));
#26502=CARTESIAN_POINT('Ctrl Pts',(7.62197014916225,5.45315318247101,-3.11162923149047));
#26503=CARTESIAN_POINT('Ctrl Pts',(7.47355913123751,5.54155404080058,-3.25437523675975));
#26504=CARTESIAN_POINT('Ctrl Pts',(7.399999514344,5.59163607462568,-3.31415314694812));
#26505=CARTESIAN_POINT('',(7.6395955992633,6.25001191701594,0.360574957917378));
#26506=CARTESIAN_POINT('Ctrl Pts',(7.63959559912056,6.2500119169745,-0.36057495784842));
#26507=CARTESIAN_POINT('Ctrl Pts',(7.66390188127962,6.22779773364639,-0.323611089501758));
#26508=CARTESIAN_POINT('Ctrl Pts',(7.6858526263557,6.20786999945922,-0.282558774022251));
#26509=CARTESIAN_POINT('Ctrl Pts',(7.73340207567264,6.16485627699069,-0.164015832549452));
#26510=CARTESIAN_POINT('Ctrl Pts',(7.75,6.15,-0.0807152191716278));
#26511=CARTESIAN_POINT('Ctrl Pts',(7.75,6.15,0.080715219171628));
#26512=CARTESIAN_POINT('Ctrl Pts',(7.73340207567264,6.16485627699069,0.164015832549452));
#26513=CARTESIAN_POINT('Ctrl Pts',(7.6858526263557,6.20786999945922,0.282558774022251));
#26514=CARTESIAN_POINT('Ctrl Pts',(7.66390188127961,6.22779773364639,0.32361108950176));
#26515=CARTESIAN_POINT('Ctrl Pts',(7.63959559912056,6.2500119169745,0.36057495784842));
#26516=CARTESIAN_POINT('Ctrl Pts',(7.4,6.43629745752619,0.907785788741997));
#26517=CARTESIAN_POINT('Ctrl Pts',(7.53289072319445,6.34140579300535,0.629043024174527));
#26518=CARTESIAN_POINT('Ctrl Pts',(7.6395955992633,6.25001191701594,0.360574957917378));
#26519=CARTESIAN_POINT('',(7.6395955992633,5.91224415060338,2.05864818917039));
#26520=CARTESIAN_POINT('Ctrl Pts',(7.6395955992633,5.91224415060338,2.05864818917039));
#26521=CARTESIAN_POINT('Ctrl Pts',(7.53289072318166,6.09941936310245,1.84559095978961));
#26522=CARTESIAN_POINT('Ctrl Pts',(7.4,6.29375806765092,1.62437969264548));
#26523=CARTESIAN_POINT('',(7.6395955992633,5.63627202556194,2.72490383628236));
#26524=CARTESIAN_POINT('Ctrl Pts',(7.63959559912056,5.91224415053871,2.05864818921824));
#26525=CARTESIAN_POINT('Ctrl Pts',(7.66390188127962,5.87757546121802,2.08429735070297));
#26526=CARTESIAN_POINT('Ctrl Pts',(7.6858526263557,5.84345459447894,2.11459873101869));
#26527=CARTESIAN_POINT('Ctrl Pts',(7.73340207567264,5.75835067694767,2.20765748941603));
#26528=CARTESIAN_POINT('Ctrl Pts',(7.75,5.71274750206111,2.27893197009047));
#26529=CARTESIAN_POINT('Ctrl Pts',(7.75,5.65097074782771,2.42807424800013));
#26530=CARTESIAN_POINT('Ctrl Pts',(7.73340207567264,5.63281839342319,2.5107192308165));
#26531=CARTESIAN_POINT('Ctrl Pts',(7.6858526263557,5.62719347150352,2.63669926711996));
#26532=CARTESIAN_POINT('Ctrl Pts',(7.66390188127962,5.62989425625414,2.68225267487168));
#26533=CARTESIAN_POINT('Ctrl Pts',(7.63959559912056,5.63627202555004,2.72490383620279));
#26534=CARTESIAN_POINT('Ctrl Pts',(7.4,5.59896890467484,3.30174911289217));
#26535=CARTESIAN_POINT('Ctrl Pts',(7.53289072319445,5.61797067590972,3.007910909991));
#26536=CARTESIAN_POINT('Ctrl Pts',(7.6395955992633,5.63627202556194,2.72490383628236));
#26537=CARTESIAN_POINT('',(7.6395955992633,4.67439080688814,4.16446081114928));
#26538=CARTESIAN_POINT('Ctrl Pts',(7.6395955992633,4.67439080688814,4.16446081114928));
#26539=CARTESIAN_POINT('Ctrl Pts',(7.53289072318166,4.92885162653911,4.03925045044362));
#26540=CARTESIAN_POINT('Ctrl Pts',(7.4,5.19305106503475,3.90924809086626));
#26541=CARTESIAN_POINT('',(7.6395955992633,4.16446081114928,4.67439080688814));
#26542=CARTESIAN_POINT('Ctrl Pts',(7.63959559912056,4.67439080681008,4.16446081116873));
#26543=CARTESIAN_POINT('Ctrl Pts',(7.66390188127962,4.63254560517343,4.17489041346571));
#26544=CARTESIAN_POINT('Ctrl Pts',(7.6858526263557,4.58942619853704,4.18982774814726));
#26545=CARTESIAN_POINT('Ctrl Pts',(7.73340207567264,4.47518838591824,4.2432349710829));
#26546=CARTESIAN_POINT('Ctrl Pts',(7.75,4.40578098311848,4.29163242547605));
#26547=CARTESIAN_POINT('Ctrl Pts',(7.75,4.29163242547605,4.40578098311848));
#26548=CARTESIAN_POINT('Ctrl Pts',(7.73340207567264,4.2432349710829,4.47518838591824));
#26549=CARTESIAN_POINT('Ctrl Pts',(7.6858526263557,4.18982774814726,4.58942619853704));
#26550=CARTESIAN_POINT('Ctrl Pts',(7.66390188127962,4.17489041346571,4.63254560517343));
#26551=CARTESIAN_POINT('Ctrl Pts',(7.63959559912056,4.16446081116873,4.67439080681008));
#26552=CARTESIAN_POINT('Ctrl Pts',(7.4,3.90924809086626,5.19305106503475));
#26553=CARTESIAN_POINT('Ctrl Pts',(7.53289072319445,4.03925045043784,4.92885162654164));
#26554=CARTESIAN_POINT('Ctrl Pts',(7.6395955992633,4.16446081114928,4.67439080688814));
#26555=CARTESIAN_POINT('',(7.6395955992633,2.72490383628236,5.63627202556194));
#26556=CARTESIAN_POINT('Ctrl Pts',(7.6395955992633,2.72490383628236,5.63627202556194));
#26557=CARTESIAN_POINT('Ctrl Pts',(7.53289072318166,3.00791090998645,5.61797067591409));
#26558=CARTESIAN_POINT('Ctrl Pts',(7.4,3.30174911289217,5.59896890467484));
#26559=CARTESIAN_POINT('',(7.6395955992633,2.05864818917039,5.91224415060338));
#26560=CARTESIAN_POINT('Ctrl Pts',(7.63959559912056,2.72490383620279,5.63627202555004));
#26561=CARTESIAN_POINT('Ctrl Pts',(7.66390188127962,2.68225267487168,5.62989425625414));
#26562=CARTESIAN_POINT('Ctrl Pts',(7.6858526263557,2.63669926711996,5.62719347150352));
#26563=CARTESIAN_POINT('Ctrl Pts',(7.73340207567264,2.5107192308165,5.63281839342319));
#26564=CARTESIAN_POINT('Ctrl Pts',(7.75,2.42807424800013,5.65097074782771));
#26565=CARTESIAN_POINT('Ctrl Pts',(7.75,2.27893197009047,5.71274750206111));
#26566=CARTESIAN_POINT('Ctrl Pts',(7.73340207567264,2.20765748941603,5.75835067694767));
#26567=CARTESIAN_POINT('Ctrl Pts',(7.6858526263557,2.11459873101869,5.84345459447894));
#26568=CARTESIAN_POINT('Ctrl Pts',(7.66390188127962,2.08429735070298,5.87757546121802));
#26569=CARTESIAN_POINT('Ctrl Pts',(7.63959559912056,2.05864818921824,5.9122441505387));
#26570=CARTESIAN_POINT('Ctrl Pts',(7.4,1.62437969264548,6.29375806765092));
#26571=CARTESIAN_POINT('Ctrl Pts',(7.53289072319445,1.8455909597833,6.09941936310257));
#26572=CARTESIAN_POINT('Ctrl Pts',(7.6395955992633,2.05864818917039,5.91224415060338));
#26573=CARTESIAN_POINT('',(7.6395955992633,0.360574957917379,6.25001191701594));
#26574=CARTESIAN_POINT('Ctrl Pts',(7.6395955992633,0.360574957917379,6.25001191701594));
#26575=CARTESIAN_POINT('Ctrl Pts',(7.53289072318166,0.629043024168653,6.34140579300765));
#26576=CARTESIAN_POINT('Ctrl Pts',(7.4,0.907785788741998,6.43629745752619));
#26577=CARTESIAN_POINT('',(7.6395955992633,-0.360574957917378,6.25001191701594));
#26578=CARTESIAN_POINT('Ctrl Pts',(7.63959559912056,0.36057495784842,6.2500119169745));
#26579=CARTESIAN_POINT('Ctrl Pts',(7.66390188127962,0.32361108950176,6.22779773364639));
#26580=CARTESIAN_POINT('Ctrl Pts',(7.6858526263557,0.282558774022251,6.20786999945922));
#26581=CARTESIAN_POINT('Ctrl Pts',(7.73340207567264,0.164015832549452,6.16485627699069));
#26582=CARTESIAN_POINT('Ctrl Pts',(7.75,0.0807152191716284,6.15));
#26583=CARTESIAN_POINT('Ctrl Pts',(7.75,-0.0807152191716275,6.15));
#26584=CARTESIAN_POINT('Ctrl Pts',(7.73340207567264,-0.16401583254945,6.16485627699069));
#26585=CARTESIAN_POINT('Ctrl Pts',(7.6858526263557,-0.282558774022249,6.20786999945922));
#26586=CARTESIAN_POINT('Ctrl Pts',(7.66390188127962,-0.323611089501759,
6.22779773364639));
#26587=CARTESIAN_POINT('Ctrl Pts',(7.63959559912056,-0.360574957848421,
6.2500119169745));
#26588=CARTESIAN_POINT('Ctrl Pts',(7.4,-0.907785788741997,6.43629745752619));
#26589=CARTESIAN_POINT('Ctrl Pts',(7.53289072319445,-0.629043024174527,
6.34140579300535));
#26590=CARTESIAN_POINT('Ctrl Pts',(7.6395955992633,-0.360574957917378,6.25001191701594));
#26591=CARTESIAN_POINT('',(7.6395955992633,-2.05864818917039,5.91224415060338));
#26592=CARTESIAN_POINT('Ctrl Pts',(7.6395955992633,-2.05864818917039,5.91224415060338));
#26593=CARTESIAN_POINT('Ctrl Pts',(7.53289072318166,-1.84559095978961,6.09941936310245));
#26594=CARTESIAN_POINT('Ctrl Pts',(7.4,-1.62437969264548,6.29375806765092));
#26595=CARTESIAN_POINT('',(7.6395955992633,-2.72490383628236,5.63627202556194));
#26596=CARTESIAN_POINT('Ctrl Pts',(7.63959559912056,-2.05864818921824,5.91224415053871));
#26597=CARTESIAN_POINT('Ctrl Pts',(7.66390188127962,-2.08429735070297,5.87757546121802));
#26598=CARTESIAN_POINT('Ctrl Pts',(7.6858526263557,-2.11459873101868,5.84345459447894));
#26599=CARTESIAN_POINT('Ctrl Pts',(7.73340207567264,-2.20765748941603,5.75835067694767));
#26600=CARTESIAN_POINT('Ctrl Pts',(7.75,-2.27893197009047,5.71274750206111));
#26601=CARTESIAN_POINT('Ctrl Pts',(7.75,-2.42807424800013,5.65097074782771));
#26602=CARTESIAN_POINT('Ctrl Pts',(7.73340207567264,-2.5107192308165,5.63281839342319));
#26603=CARTESIAN_POINT('Ctrl Pts',(7.6858526263557,-2.63669926711996,5.62719347150352));
#26604=CARTESIAN_POINT('Ctrl Pts',(7.66390188127962,-2.68225267487168,5.62989425625414));
#26605=CARTESIAN_POINT('Ctrl Pts',(7.63959559912056,-2.72490383620279,5.63627202555004));
#26606=CARTESIAN_POINT('Ctrl Pts',(7.4,-3.30174911289217,5.59896890467484));
#26607=CARTESIAN_POINT('Ctrl Pts',(7.53289072319445,-3.007910909991,5.61797067590973));
#26608=CARTESIAN_POINT('Ctrl Pts',(7.6395955992633,-2.72490383628236,5.63627202556194));
#26609=CARTESIAN_POINT('',(7.6395955992633,-4.16446081114928,4.67439080688814));
#26610=CARTESIAN_POINT('Ctrl Pts',(7.6395955992633,-4.16446081114928,4.67439080688814));
#26611=CARTESIAN_POINT('Ctrl Pts',(7.53289072318166,-4.03925045044361,4.92885162653911));
#26612=CARTESIAN_POINT('Ctrl Pts',(7.4,-3.90924809086626,5.19305106503475));
#26613=CARTESIAN_POINT('',(7.6395955992633,-4.67439080688814,4.16446081114928));
#26614=CARTESIAN_POINT('Ctrl Pts',(7.63959559912056,-4.16446081116873,4.67439080681008));
#26615=CARTESIAN_POINT('Ctrl Pts',(7.66390188127962,-4.17489041346571,4.63254560517343));
#26616=CARTESIAN_POINT('Ctrl Pts',(7.6858526263557,-4.18982774814726,4.58942619853704));
#26617=CARTESIAN_POINT('Ctrl Pts',(7.73340207567264,-4.2432349710829,4.47518838591824));
#26618=CARTESIAN_POINT('Ctrl Pts',(7.75,-4.29163242547605,4.40578098311848));
#26619=CARTESIAN_POINT('Ctrl Pts',(7.75,-4.40578098311848,4.29163242547605));
#26620=CARTESIAN_POINT('Ctrl Pts',(7.73340207567264,-4.47518838591824,4.2432349710829));
#26621=CARTESIAN_POINT('Ctrl Pts',(7.6858526263557,-4.58942619853704,4.18982774814726));
#26622=CARTESIAN_POINT('Ctrl Pts',(7.66390188127962,-4.63254560517344,4.17489041346571));
#26623=CARTESIAN_POINT('Ctrl Pts',(7.63959559912056,-4.67439080681008,4.16446081116873));
#26624=CARTESIAN_POINT('Ctrl Pts',(7.4,-5.19305106503475,3.90924809086626));
#26625=CARTESIAN_POINT('Ctrl Pts',(7.53289072319445,-4.92885162654164,4.03925045043784));
#26626=CARTESIAN_POINT('Ctrl Pts',(7.6395955992633,-4.67439080688814,4.16446081114927));
#26627=CARTESIAN_POINT('',(7.6395955992633,-5.63627202556194,2.72490383628236));
#26628=CARTESIAN_POINT('Ctrl Pts',(7.6395955992633,-5.63627202556194,2.72490383628236));
#26629=CARTESIAN_POINT('Ctrl Pts',(7.53289072318166,-5.61797067591409,3.00791090998645));
#26630=CARTESIAN_POINT('Ctrl Pts',(7.4,-5.59896890467484,3.30174911289217));
#26631=CARTESIAN_POINT('',(7.6395955992633,-5.91224415060338,2.05864818917039));
#26632=CARTESIAN_POINT('Ctrl Pts',(7.63959559912056,-5.63627202555004,2.72490383620279));
#26633=CARTESIAN_POINT('Ctrl Pts',(7.66390188127962,-5.62989425625414,2.68225267487168));
#26634=CARTESIAN_POINT('Ctrl Pts',(7.6858526263557,-5.62719347150352,2.63669926711996));
#26635=CARTESIAN_POINT('Ctrl Pts',(7.73340207567264,-5.63281839342319,2.5107192308165));
#26636=CARTESIAN_POINT('Ctrl Pts',(7.75,-5.65097074782771,2.42807424800013));
#26637=CARTESIAN_POINT('Ctrl Pts',(7.75,-5.71274750206111,2.27893197009047));
#26638=CARTESIAN_POINT('Ctrl Pts',(7.73340207567264,-5.75835067694767,2.20765748941603));
#26639=CARTESIAN_POINT('Ctrl Pts',(7.6858526263557,-5.84345459447894,2.11459873101869));
#26640=CARTESIAN_POINT('Ctrl Pts',(7.66390188127962,-5.87757546121802,2.08429735070297));
#26641=CARTESIAN_POINT('Ctrl Pts',(7.63959559912056,-5.91224415053871,2.05864818921824));
#26642=CARTESIAN_POINT('Ctrl Pts',(7.4,-6.29375806765092,1.62437969264548));
#26643=CARTESIAN_POINT('Ctrl Pts',(7.53289072319445,-6.09941936310258,1.8455909597833));
#26644=CARTESIAN_POINT('Ctrl Pts',(7.6395955992633,-5.91224415060338,2.05864818917039));
#26645=CARTESIAN_POINT('',(7.6395955992633,-6.25001191701594,0.360574957917379));
#26646=CARTESIAN_POINT('Ctrl Pts',(7.6395955992633,-6.25001191701594,0.360574957917379));
#26647=CARTESIAN_POINT('Ctrl Pts',(7.53289072318166,-6.34140579300764,0.629043024168652));
#26648=CARTESIAN_POINT('Ctrl Pts',(7.4,-6.43629745752619,0.907785788741998));
#26649=CARTESIAN_POINT('Ctrl Pts',(7.63959559912056,-6.2500119169745,0.360574957848422));
#26650=CARTESIAN_POINT('Ctrl Pts',(7.66390188127962,-6.22779773364639,0.32361108950176));
#26651=CARTESIAN_POINT('Ctrl Pts',(7.6858526263557,-6.20786999945922,0.282558774022252));
#26652=CARTESIAN_POINT('Ctrl Pts',(7.73340207567264,-6.16485627699069,0.164015832549452));
#26653=CARTESIAN_POINT('Ctrl Pts',(7.75,-6.15,0.0807152191716289));
#26654=CARTESIAN_POINT('Ctrl Pts',(7.75,-6.15,9.28077059647592E-16));
#26655=CARTESIAN_POINT('Origin',(3.95,6.34315468735702,0.634180373472705));
#26656=CARTESIAN_POINT('',(0.6,6.25001191718784,0.360574958203413));
#26657=CARTESIAN_POINT('',(3.95,6.25001191718784,0.360574958203413));
#26658=CARTESIAN_POINT('',(0.6,6.2727384556044,0.427333805613703));
#26659=CARTESIAN_POINT('Origin',(3.95,6.10300110926129,1.84151394080869));
#26660=CARTESIAN_POINT('',(0.6,5.91224415087166,2.05864818897191));
#26661=CARTESIAN_POINT('',(0.6,5.95878823942725,2.00566812596253));
#26662=CARTESIAN_POINT('',(3.95,5.91224415087166,2.05864818897191));
#26663=CARTESIAN_POINT('Origin',(3.95,5.61762046514307,3.01332647475229));
#26664=CARTESIAN_POINT('',(0.6,5.63627202561129,2.72490383661241));
#26665=CARTESIAN_POINT('',(3.95,5.63627202561129,2.72490383661241));
#26666=CARTESIAN_POINT('',(0.6,5.63172110443148,2.79527803907584));
#26667=CARTESIAN_POINT('Origin',(3.95,4.93372093612335,4.03685445096741));
#26668=CARTESIAN_POINT('',(0.6,4.67439080721195,4.16446081106857));
#26669=CARTESIAN_POINT('',(0.6,4.73766653034721,4.1333252667878));
#26670=CARTESIAN_POINT('',(3.95,4.67439080721195,4.16446081106857));
#26671=CARTESIAN_POINT('Origin',(3.95,4.03685445096741,4.93372093612335));
#26672=CARTESIAN_POINT('',(0.6,4.16446081106857,4.67439080721195));
#26673=CARTESIAN_POINT('',(3.95,4.16446081106857,4.67439080721195));
#26674=CARTESIAN_POINT('',(0.6,4.1333252667878,4.73766653034721));
#26675=CARTESIAN_POINT('Origin',(3.95,3.01332647475228,5.61762046514307));
#26676=CARTESIAN_POINT('',(0.6,2.7249038366124,5.63627202561129));
#26677=CARTESIAN_POINT('',(0.6,2.79527803907584,5.63172110443148));
#26678=CARTESIAN_POINT('',(3.95,2.7249038366124,5.63627202561129));
#26679=CARTESIAN_POINT('Origin',(3.95,1.8415139408087,6.10300110926129));
#26680=CARTESIAN_POINT('',(0.6,2.05864818897191,5.91224415087166));
#26681=CARTESIAN_POINT('',(3.95,2.05864818897191,5.91224415087166));
#26682=CARTESIAN_POINT('',(0.6,2.00566812596253,5.95878823942725));
#26683=CARTESIAN_POINT('Origin',(3.95,0.634180373472706,6.34315468735702));
#26684=CARTESIAN_POINT('',(0.6,0.360574958203414,6.25001191718784));
#26685=CARTESIAN_POINT('',(0.6,0.427333805613703,6.2727384556044));
#26686=CARTESIAN_POINT('',(3.95,0.360574958203414,6.25001191718784));
#26687=CARTESIAN_POINT('Origin',(3.95,-0.634180373472705,6.34315468735702));
#26688=CARTESIAN_POINT('',(0.6,-0.360574958203413,6.25001191718784));
#26689=CARTESIAN_POINT('',(3.95,-0.360574958203413,6.25001191718784));
#26690=CARTESIAN_POINT('',(0.6,-0.427333805613702,6.2727384556044));
#26691=CARTESIAN_POINT('Origin',(3.95,-1.84151394080869,6.10300110926129));
#26692=CARTESIAN_POINT('',(0.6,-2.05864818897191,5.91224415087166));
#26693=CARTESIAN_POINT('',(0.6,-2.00566812596253,5.95878823942725));
#26694=CARTESIAN_POINT('',(3.95,-2.05864818897191,5.91224415087166));
#26695=CARTESIAN_POINT('Origin',(3.95,-3.01332647475229,5.61762046514307));
#26696=CARTESIAN_POINT('',(0.6,-2.7249038366124,5.63627202561129));
#26697=CARTESIAN_POINT('',(3.95,-2.7249038366124,5.63627202561129));
#26698=CARTESIAN_POINT('',(0.6,-2.79527803907584,5.63172110443148));
#26699=CARTESIAN_POINT('Origin',(3.95,-4.03685445096741,4.93372093612335));
#26700=CARTESIAN_POINT('',(0.6,-4.16446081106857,4.67439080721195));
#26701=CARTESIAN_POINT('',(0.6,-4.1333252667878,4.73766653034721));
#26702=CARTESIAN_POINT('',(3.95,-4.16446081106857,4.67439080721195));
#26703=CARTESIAN_POINT('Origin',(3.95,-4.93372093612335,4.03685445096741));
#26704=CARTESIAN_POINT('',(0.6,-4.67439080721195,4.16446081106857));
#26705=CARTESIAN_POINT('',(3.95,-4.67439080721195,4.16446081106857));
#26706=CARTESIAN_POINT('',(0.6,-4.73766653034721,4.1333252667878));
#26707=CARTESIAN_POINT('Origin',(3.95,-5.61762046514307,3.01332647475228));
#26708=CARTESIAN_POINT('',(0.6,-5.63627202561129,2.7249038366124));
#26709=CARTESIAN_POINT('',(0.6,-5.63172110443148,2.79527803907584));
#26710=CARTESIAN_POINT('',(3.95,-5.63627202561129,2.7249038366124));
#26711=CARTESIAN_POINT('Origin',(3.95,-6.10300110926129,1.8415139408087));
#26712=CARTESIAN_POINT('',(0.6,-5.91224415087166,2.05864818897191));
#26713=CARTESIAN_POINT('',(3.95,-5.91224415087166,2.05864818897191));
#26714=CARTESIAN_POINT('',(0.6,-5.95878823942725,2.00566812596253));
#26715=CARTESIAN_POINT('Origin',(3.95,-6.34315468735702,0.634180373472706));
#26716=CARTESIAN_POINT('',(0.6,-6.25001191718784,0.360574958203414));
#26717=CARTESIAN_POINT('',(0.6,-6.2727384556044,0.427333805613704));
#26718=CARTESIAN_POINT('',(3.95,-6.25001191718784,0.360574958203414));
#26719=CARTESIAN_POINT('Origin',(3.95,-6.34315468735702,-0.634180373472705));
#26720=CARTESIAN_POINT('',(0.6,-6.25001191718784,-0.360574958203412));
#26721=CARTESIAN_POINT('',(3.95,-6.25001191718784,-0.360574958203413));
#26722=CARTESIAN_POINT('',(0.6,-6.2727384556044,-0.427333805613702));
#26723=CARTESIAN_POINT('Origin',(3.95,-6.10300110926129,-1.84151394080869));
#26724=CARTESIAN_POINT('',(0.6,-5.91224415087166,-2.05864818897191));
#26725=CARTESIAN_POINT('',(0.6,-5.95878823942725,-2.00566812596253));
#26726=CARTESIAN_POINT('',(3.95,-5.91224415087166,-2.05864818897191));
#26727=CARTESIAN_POINT('Origin',(3.95,-5.61762046514307,-3.01332647475229));
#26728=CARTESIAN_POINT('',(0.6,-5.6362720256113,-2.7249038366124));
#26729=CARTESIAN_POINT('',(3.95,-5.6362720256113,-2.7249038366124));
#26730=CARTESIAN_POINT('',(0.6,-5.63172110443148,-2.79527803907584));
#26731=CARTESIAN_POINT('Origin',(3.95,-4.93372093612335,-4.03685445096742));
#26732=CARTESIAN_POINT('',(0.6,-4.67439080721195,-4.16446081106857));
#26733=CARTESIAN_POINT('',(0.6,-4.73766653034721,-4.1333252667878));
#26734=CARTESIAN_POINT('',(3.95,-4.67439080721195,-4.16446081106857));
#26735=CARTESIAN_POINT('Origin',(3.95,-4.03685445096742,-4.93372093612334));
#26736=CARTESIAN_POINT('',(0.6,-4.16446081106857,-4.67439080721194));
#26737=CARTESIAN_POINT('',(3.95,-4.16446081106857,-4.67439080721194));
#26738=CARTESIAN_POINT('',(0.6,-4.1333252667878,-4.73766653034721));
#26739=CARTESIAN_POINT('Origin',(3.95,-3.01332647475229,-5.61762046514307));
#26740=CARTESIAN_POINT('',(0.6,-2.72490383661241,-5.63627202561129));
#26741=CARTESIAN_POINT('',(0.6,-2.79527803907584,-5.63172110443147));
#26742=CARTESIAN_POINT('',(3.95,-2.72490383661241,-5.63627202561129));
#26743=CARTESIAN_POINT('Origin',(3.95,-1.8415139408087,-6.10300110926129));
#26744=CARTESIAN_POINT('',(0.6,-2.05864818897192,-5.91224415087166));
#26745=CARTESIAN_POINT('',(3.95,-2.05864818897192,-5.91224415087166));
#26746=CARTESIAN_POINT('',(0.6,-2.00566812596253,-5.95878823942725));
#26747=CARTESIAN_POINT('Origin',(3.95,-0.634180373472707,-6.34315468735702));
#26748=CARTESIAN_POINT('',(0.6,-0.360574958203415,-6.25001191718784));
#26749=CARTESIAN_POINT('',(0.6,-0.427333805613704,-6.2727384556044));
#26750=CARTESIAN_POINT('',(3.95,-0.360574958203415,-6.25001191718784));
#26751=CARTESIAN_POINT('Origin',(3.95,0.634180373472704,-6.34315468735702));
#26752=CARTESIAN_POINT('',(0.6,0.360574958203412,-6.25001191718784));
#26753=CARTESIAN_POINT('',(3.95,0.360574958203412,-6.25001191718784));
#26754=CARTESIAN_POINT('',(0.6,0.427333805613702,-6.2727384556044));
#26755=CARTESIAN_POINT('Origin',(3.95,1.8415139408087,-6.10300110926129));
#26756=CARTESIAN_POINT('',(0.6,2.05864818897191,-5.91224415087166));
#26757=CARTESIAN_POINT('',(0.6,2.00566812596253,-5.95878823942725));
#26758=CARTESIAN_POINT('',(3.95,2.05864818897191,-5.91224415087166));
#26759=CARTESIAN_POINT('Origin',(3.95,3.01332647475229,-5.61762046514307));
#26760=CARTESIAN_POINT('',(0.6,2.72490383661241,-5.63627202561129));
#26761=CARTESIAN_POINT('',(3.95,2.72490383661241,-5.63627202561129));
#26762=CARTESIAN_POINT('',(0.6,2.79527803907584,-5.63172110443148));
#26763=CARTESIAN_POINT('Origin',(3.95,4.03685445096741,-4.93372093612335));
#26764=CARTESIAN_POINT('',(0.6,4.16446081106857,-4.67439080721195));
#26765=CARTESIAN_POINT('',(0.6,4.1333252667878,-4.73766653034721));
#26766=CARTESIAN_POINT('',(3.95,4.16446081106857,-4.67439080721195));
#26767=CARTESIAN_POINT('Origin',(3.95,4.93372093612335,-4.03685445096741));
#26768=CARTESIAN_POINT('',(0.6,4.67439080721195,-4.16446081106857));
#26769=CARTESIAN_POINT('',(3.95,4.67439080721195,-4.16446081106857));
#26770=CARTESIAN_POINT('',(0.6,4.7376665303472,-4.1333252667878));
#26771=CARTESIAN_POINT('Ctrl Pts',(7.39428617940509,5.5955384738582,-3.31877409641756));
#26772=CARTESIAN_POINT('Ctrl Pts',(7.46976289566289,5.54381939543681,-3.25801858335938));
#26773=CARTESIAN_POINT('Ctrl Pts',(7.62033583663474,5.45380336720261,-3.11382584884576));
#26774=CARTESIAN_POINT('Ctrl Pts',(7.81463329279646,5.37650527564507,-2.85267802239966));
#26775=CARTESIAN_POINT('Ctrl Pts',(7.98425119443302,5.38246983194813,-2.46771855869631));
#26776=CARTESIAN_POINT('Ctrl Pts',(7.97308777074854,5.61920950447284,-1.91938073772091));
#26777=CARTESIAN_POINT('Ctrl Pts',(7.67997347882042,5.99409705965181,-1.66087268674238));
#26778=CARTESIAN_POINT('Ctrl Pts',(7.4697628956628,6.22383932171217,-1.61630525466166));
#26779=CARTESIAN_POINT('Ctrl Pts',(7.394286179405,6.30337086805857,-1.60991553045225));
#26780=CARTESIAN_POINT('Ctrl Pts',(7.29765887109684,5.62436223494091,-3.17572382553274));
#26781=CARTESIAN_POINT('Ctrl Pts',(7.36647595579574,5.5822650494995,-3.11685834537302));
#26782=CARTESIAN_POINT('Ctrl Pts',(7.501350054236,5.5120996672264,-2.98212215980868));
#26783=CARTESIAN_POINT('Ctrl Pts',(7.66846140186336,5.45952849244207,-2.75326447440463));
#26784=CARTESIAN_POINT('Ctrl Pts',(7.80024313771858,5.47482631338047,-2.44676755506769));
#26785=CARTESIAN_POINT('Ctrl Pts',(7.79287204927538,5.65171340584687,-2.03492319836375));
#26786=CARTESIAN_POINT('Ctrl Pts',(7.55870439802978,5.9466451212402,-1.80165889219619));
#26787=CARTESIAN_POINT('Ctrl Pts',(7.36647595579565,6.15120914289298,-1.7433057988706));
#26788=CARTESIAN_POINT('Ctrl Pts',(7.29765887109675,6.22260052838622,-1.73144882396635));
#26789=CARTESIAN_POINT('Ctrl Pts',(7.20103156278858,5.65318599602361,-3.03267355464793));
#26790=CARTESIAN_POINT('Ctrl Pts',(7.26318901592858,5.62071070356219,-2.97569810738666));
#26791=CARTESIAN_POINT('Ctrl Pts',(7.38236427183726,5.57039596725019,-2.8504184707716));
#26792=CARTESIAN_POINT('Ctrl Pts',(7.52228951093026,5.54255170923908,-2.6538509264096));
#26793=CARTESIAN_POINT('Ctrl Pts',(7.61623508100414,5.56718279481282,-2.42581655143907));
#26794=CARTESIAN_POINT('Ctrl Pts',(7.61265632780222,5.6842173072209,-2.15046565900658));
#26795=CARTESIAN_POINT('Ctrl Pts',(7.43743531723913,5.89919318282859,-1.94244509765));
#26796=CARTESIAN_POINT('Ctrl Pts',(7.26318901592851,6.07857896407379,-1.87030634307954));
#26797=CARTESIAN_POINT('Ctrl Pts',(7.2010315627885,6.14183018871386,-1.85298211748045));
#26798=CARTESIAN_POINT('Ctrl Pts',(7.10440425448033,5.68200975710631,-2.88962328376311));
#26799=CARTESIAN_POINT('Ctrl Pts',(7.15990207606142,5.65915635762488,-2.8345378694003));
#26800=CARTESIAN_POINT('Ctrl Pts',(7.26337848943852,5.62869226727397,-2.71871478173452));
#26801=CARTESIAN_POINT('Ctrl Pts',(7.37611761999717,5.62557492603609,-2.55443737841458));
#26802=CARTESIAN_POINT('Ctrl Pts',(7.43222702428969,5.65953927624516,-2.40486554781045));
#26803=CARTESIAN_POINT('Ctrl Pts',(7.43244060632906,5.71672120859493,-2.26600811964941));
#26804=CARTESIAN_POINT('Ctrl Pts',(7.31616623644848,5.85174124441698,-2.08323130310381));
#26805=CARTESIAN_POINT('Ctrl Pts',(7.15990207606136,6.0059487852546,-1.99730688728848));
#26806=CARTESIAN_POINT('Ctrl Pts',(7.10440425448025,6.06105984904151,-1.97451541099454));
#26807=CARTESIAN_POINT('',(7.25292710453826,5.63627202561129,-2.72490383661241));
#26808=CARTESIAN_POINT('',(7.25292710453827,5.91224415087166,-2.05864818897192));
#26809=CARTESIAN_POINT('Ctrl Pts',(7.25269877985884,5.63645713070299,-2.72481700882979));
#26810=CARTESIAN_POINT('Ctrl Pts',(7.25390396092312,5.6362292427284,-2.72330726216592));
#26811=CARTESIAN_POINT('Ctrl Pts',(7.29995254002791,5.62768096094605,-2.66542104042265));
#26812=CARTESIAN_POINT('Ctrl Pts',(7.37611761999717,5.62557492603609,-2.55443737841458));
#26813=CARTESIAN_POINT('Ctrl Pts',(7.43222702428969,5.65953927624516,-2.40486554781045));
#26814=CARTESIAN_POINT('Ctrl Pts',(7.43244060632906,5.71672120859493,-2.26600811964941));
#26815=CARTESIAN_POINT('Ctrl Pts',(7.3444569328455,5.81888954335097,-2.12770269805194));
#26816=CARTESIAN_POINT('Ctrl Pts',(7.25402238610438,5.91146676762003,-2.0584409850931));
#26817=CARTESIAN_POINT('Ctrl Pts',(7.25282290367468,5.91269329897841,-2.05753054923321));
#26818=CARTESIAN_POINT('Ctrl Pts',(7.25292710457906,5.91224415071533,-2.05864818914986));
#26819=CARTESIAN_POINT('Ctrl Pts',(7.2457805786392,5.93962960438486,-2.0274759585621));
#26820=CARTESIAN_POINT('Ctrl Pts',(7.24511949066774,5.96740428223051,-1.99586068306754));
#26821=CARTESIAN_POINT('Ctrl Pts',(7.25392829017846,6.03832444366435,-1.91513389824904));
#26822=CARTESIAN_POINT('Ctrl Pts',(7.2698369054514,6.08532226073065,-1.86163736653582));
#26823=CARTESIAN_POINT('Ctrl Pts',(7.31848027241684,6.18902485431357,-1.74359509494429));
#26824=CARTESIAN_POINT('Ctrl Pts',(7.35068643968617,6.24363465640856,-1.68143401615411));
#26825=CARTESIAN_POINT('Ctrl Pts',(7.38278617788903,6.2937580676509,-1.6243796926455));
#26826=CARTESIAN_POINT('Ctrl Pts',(7.38278617788903,5.59896890467484,-3.30174911289214));
#26827=CARTESIAN_POINT('Ctrl Pts',(7.36731678113116,5.6013307273702,-3.26522653164345));
#26828=CARTESIAN_POINT('Ctrl Pts',(7.35173106112422,5.60381146615418,-3.22690841479602));
#26829=CARTESIAN_POINT('Ctrl Pts',(7.33695451365628,5.60633295692038,-3.18798774492175));
#26830=CARTESIAN_POINT('Ctrl Pts',(7.32259692411982,5.60878295611807,-3.15017058879979));
#26831=CARTESIAN_POINT('Ctrl Pts',(7.30900069055514,5.61127616857016,-3.11178444084887));
#26832=CARTESIAN_POINT('Ctrl Pts',(7.2969989223891,5.61374501140461,-3.07394552961325));
#26833=CARTESIAN_POINT('Ctrl Pts',(7.29357288432376,5.61444977002109,-3.06314399200224));
#26834=CARTESIAN_POINT('Ctrl Pts',(7.29027681897695,5.61515230894107,-3.05238718446692));
#26835=CARTESIAN_POINT('Ctrl Pts',(7.28713040024107,5.61585016846552,-3.04170135195279));
#26836=CARTESIAN_POINT('Ctrl Pts',(7.27893276765674,5.61766836129272,-3.01386064282861));
#26837=CARTESIAN_POINT('Ctrl Pts',(7.27135734706788,5.61954609460126,-2.98524259075305));
#26838=CARTESIAN_POINT('Ctrl Pts',(7.26502754488307,5.62143232079745,-2.9564658321727));
#26839=CARTESIAN_POINT('Ctrl Pts',(7.26120721380904,5.62257074635002,-2.93909771515981));
#26840=CARTESIAN_POINT('Ctrl Pts',(7.25783974476678,5.62371308308983,-2.92167233545939));
#26841=CARTESIAN_POINT('Ctrl Pts',(7.25505700589891,5.62484873636172,-2.90433061300932));
#26842=CARTESIAN_POINT('Ctrl Pts',(7.25030000552081,5.62679009819994,-2.87468551004808));
#26843=CARTESIAN_POINT('Ctrl Pts',(7.24751313230281,5.62860295175123,-2.8470768605835));
#26844=CARTESIAN_POINT('Ctrl Pts',(7.24659919942187,5.63028834819705,-2.82113721885073));
#26845=CARTESIAN_POINT('Ctrl Pts',(7.2457555035245,5.6318442196362,-2.79719107382705));
#26846=CARTESIAN_POINT('Ctrl Pts',(7.24650820132933,5.63329170331371,-2.77466707014329));
#26847=CARTESIAN_POINT('Ctrl Pts',(7.24874445844377,5.63465189072976,-2.75328833157376));
#26848=CARTESIAN_POINT('Ctrl Pts',(7.24976108840657,5.63527024864274,-2.74356929432347));
#26849=CARTESIAN_POINT('Ctrl Pts',(7.25108378598209,5.63587083484386,-2.7340871419125));
#26850=CARTESIAN_POINT('Ctrl Pts',(7.25269878003204,5.63645713067024,-2.72481700861281));
#26851=CARTESIAN_POINT('Origin',(3.95,6.10300110926129,-1.8415139408087));
#26852=CARTESIAN_POINT('',(0.6,5.91224415087166,-2.05864818897192));
#26853=CARTESIAN_POINT('',(3.95,5.91224415087166,-2.05864818897192));
#26854=CARTESIAN_POINT('',(0.6,5.95878823942725,-2.00566812596253));
#26855=CARTESIAN_POINT('Origin',(3.95,5.61762046514307,-3.01332647475229));
#26856=CARTESIAN_POINT('',(0.6,5.63627202561129,-2.72490383661241));
#26857=CARTESIAN_POINT('',(0.6,5.63172110443147,-2.79527803907584));
#26858=CARTESIAN_POINT('',(3.95,5.63627202561129,-2.72490383661241));
#26859=CARTESIAN_POINT('Origin',(0.6,6.32857479770231,-2.62138151170087));
#26860=CARTESIAN_POINT('Origin',(0.6,6.32857479770231,-2.62138151170087));
#26861=CARTESIAN_POINT('Origin',(3.16,0.,0.));
#26862=CARTESIAN_POINT('',(3.,-2.47,3.02487759389396E-16));
#26863=CARTESIAN_POINT('',(3.16,-2.31,-2.82893410603039E-16));
#26864=CARTESIAN_POINT('Origin',(3.,0.,0.));
#26865=CARTESIAN_POINT('Origin',(3.,0.,0.));
#26866=CARTESIAN_POINT('',(3.,3.55,-2.04959345562317));
#26867=CARTESIAN_POINT('',(3.,3.55,2.04959345562317));
#26868=CARTESIAN_POINT('',(3.,3.55,-2.04959345562317));
#26869=CARTESIAN_POINT('',(3.,-5.55111512312578E-16,-4.09918691124634));
#26870=CARTESIAN_POINT('',(3.,-7.53008419494684E-16,-4.09918691124634));
#26871=CARTESIAN_POINT('',(3.,-3.55,-2.04959345562317));
#26872=CARTESIAN_POINT('',(3.,-3.55,-2.04959345562317));
#26873=CARTESIAN_POINT('',(3.,-3.55,2.04959345562317));
#26874=CARTESIAN_POINT('',(3.,-3.55,2.04959345562317));
#26875=CARTESIAN_POINT('',(3.,0.,4.09918691124634));
#26876=CARTESIAN_POINT('',(3.,2.51002806498228E-16,4.09918691124634));
#26877=CARTESIAN_POINT('',(3.,3.55,2.04959345562317));
#26878=CARTESIAN_POINT('Origin',(0.16,1.2825,5.02439071762272));
#26879=CARTESIAN_POINT('',(0.,-3.87,2.23434554176385));
#26880=CARTESIAN_POINT('',(0.,-1.11022302462516E-15,4.4686910835277));
#26881=CARTESIAN_POINT('',(0.,1.2025,5.16295478222823));
#26882=CARTESIAN_POINT('',(0.32,2.51002806498228E-16,4.09918691124634));
#26883=CARTESIAN_POINT('',(0.,-1.11022302462516E-15,4.4686910835277));
#26884=CARTESIAN_POINT('',(0.32,-3.55,2.04959345562317));
#26885=CARTESIAN_POINT('',(0.32,1.3625,4.88582665301721));
#26886=CARTESIAN_POINT('',(0.,-3.87,2.23434554176385));
#26887=CARTESIAN_POINT('Origin',(0.16,4.9925,1.40151777845782));
#26888=CARTESIAN_POINT('',(0.,3.87,2.23434554176385));
#26889=CARTESIAN_POINT('',(0.,5.0725,1.54008184306333));
#26890=CARTESIAN_POINT('',(0.32,3.55,2.04959345562317));
#26891=CARTESIAN_POINT('',(0.,3.87,2.23434554176385));
#26892=CARTESIAN_POINT('',(0.32,4.9125,1.26295371385231));
#26893=CARTESIAN_POINT('Origin',(0.16,3.2175,-2.4263145062694));
#26894=CARTESIAN_POINT('',(0.,3.87,-2.23434554176385));
#26895=CARTESIAN_POINT('',(0.,-2.98372437868011E-15,-4.4686910835277));
#26896=CARTESIAN_POINT('',(0.,3.2975,-2.56487857087491));
#26897=CARTESIAN_POINT('',(0.32,-7.53008419494684E-16,-4.09918691124634));
#26898=CARTESIAN_POINT('',(0.,-3.2612801348364E-15,-4.4686910835277));
#26899=CARTESIAN_POINT('',(0.32,3.55,-2.04959345562317));
#26900=CARTESIAN_POINT('',(0.32,3.1375,-2.28775044166389));
#26901=CARTESIAN_POINT('',(0.32,3.55,-2.04959345562317));
#26902=CARTESIAN_POINT('Origin',(0.16,-0.492500000000001,-3.99959398981113));
#26903=CARTESIAN_POINT('',(0.32,-3.55,-2.04959345562317));
#26904=CARTESIAN_POINT('',(0.32,-0.4125,-3.86102992520562));
#26905=CARTESIAN_POINT('',(0.,-3.87,-2.23434554176385));
#26906=CARTESIAN_POINT('',(0.,-0.572500000000001,-4.13815805441664));
#26907=CARTESIAN_POINT('',(0.,-3.87,-2.23434554176385));
#26908=CARTESIAN_POINT('Origin',(0.16,3.71,-1.02479672781159));
#26909=CARTESIAN_POINT('',(0.,3.87,-1.02479672781159));
#26910=CARTESIAN_POINT('',(0.32,3.55,-1.02479672781159));
#26911=CARTESIAN_POINT('Origin',(0.16,-3.71,1.02479672781158));
#26912=CARTESIAN_POINT('',(0.32,-3.55,1.02479672781158));
#26913=CARTESIAN_POINT('',(0.,-3.87,1.02479672781158));
#26914=CARTESIAN_POINT('Origin',(0.,3.55,2.04959345562317));
#26915=CARTESIAN_POINT('',(0.,3.55,2.04959345562317));
#26916=CARTESIAN_POINT('',(0.,2.51002806498228E-16,4.09918691124634));
#26917=CARTESIAN_POINT('Origin',(0.,3.55,-2.04959345562317));
#26918=CARTESIAN_POINT('',(0.,3.55,-2.04959345562317));
#26919=CARTESIAN_POINT('Origin',(0.,-7.53008419494684E-16,-4.09918691124634));
#26920=CARTESIAN_POINT('',(0.,-7.53008419494684E-16,-4.09918691124634));
#26921=CARTESIAN_POINT('Origin',(0.,6.,0.));
#26922=CARTESIAN_POINT('',(-6.93889390390723E-17,-6.,-7.34788079488412E-16));
#26923=CARTESIAN_POINT('Origin',(0.,0.,0.));
#26924=CARTESIAN_POINT('Origin',(0.,-3.55,-2.04959345562317));
#26925=CARTESIAN_POINT('',(0.,-3.55,-2.04959345562317));
#26926=CARTESIAN_POINT('Origin',(0.,-3.55,2.04959345562317));
#26927=CARTESIAN_POINT('',(0.,-3.55,2.04959345562317));
#26928=CARTESIAN_POINT('Origin',(0.,2.51002806498228E-16,4.09918691124634));
#26929=CARTESIAN_POINT('Origin',(0.6,6.32857479770231,-2.62138151170087));
#26930=CARTESIAN_POINT('Origin',(0.6,4.84368145112785,-4.84368145112785));
#26931=CARTESIAN_POINT('Origin',(0.6,4.84368145112785,-4.84368145112785));
#26932=CARTESIAN_POINT('Origin',(0.6,4.84368145112785,-4.84368145112785));
#26933=CARTESIAN_POINT('Origin',(0.6,2.62138151170087,-6.32857479770231));
#26934=CARTESIAN_POINT('Origin',(0.6,2.62138151170087,-6.32857479770231));
#26935=CARTESIAN_POINT('Origin',(0.6,2.62138151170087,-6.32857479770231));
#26936=CARTESIAN_POINT('Origin',(0.6,-1.25832458612391E-15,-6.85));
#26937=CARTESIAN_POINT('Origin',(0.6,-1.25832458612391E-15,-6.85));
#26938=CARTESIAN_POINT('Origin',(0.6,-1.25832458612391E-15,-6.85));
#26939=CARTESIAN_POINT('Origin',(0.6,-2.62138151170087,-6.32857479770231));
#26940=CARTESIAN_POINT('Origin',(0.6,-2.62138151170087,-6.32857479770231));
#26941=CARTESIAN_POINT('Origin',(0.6,-2.62138151170087,-6.32857479770231));
#26942=CARTESIAN_POINT('Origin',(0.6,-4.84368145112785,-4.84368145112785));
#26943=CARTESIAN_POINT('Origin',(0.6,-4.84368145112785,-4.84368145112785));
#26944=CARTESIAN_POINT('Origin',(0.6,-4.84368145112785,-4.84368145112785));
#26945=CARTESIAN_POINT('Origin',(0.6,-6.32857479770231,-2.62138151170086));
#26946=CARTESIAN_POINT('Origin',(0.6,-6.32857479770231,-2.62138151170086));
#26947=CARTESIAN_POINT('Origin',(0.6,-6.32857479770231,-2.62138151170086));
#26948=CARTESIAN_POINT('Origin',(0.6,-6.85,8.38883057415937E-16));
#26949=CARTESIAN_POINT('Origin',(0.6,-6.85,8.38883057415937E-16));
#26950=CARTESIAN_POINT('Origin',(0.6,-6.85,8.38883057415937E-16));
#26951=CARTESIAN_POINT('Origin',(0.6,-6.32857479770231,2.62138151170087));
#26952=CARTESIAN_POINT('Origin',(0.6,-6.32857479770231,2.62138151170087));
#26953=CARTESIAN_POINT('Origin',(0.6,-6.32857479770231,2.62138151170087));
#26954=CARTESIAN_POINT('Origin',(0.6,-4.84368145112785,4.84368145112785));
#26955=CARTESIAN_POINT('Origin',(0.6,-4.84368145112785,4.84368145112785));
#26956=CARTESIAN_POINT('Origin',(0.6,-4.84368145112785,4.84368145112785));
#26957=CARTESIAN_POINT('Origin',(0.6,-2.62138151170086,6.32857479770231));
#26958=CARTESIAN_POINT('Origin',(0.6,-2.62138151170086,6.32857479770231));
#26959=CARTESIAN_POINT('Origin',(0.6,-2.62138151170086,6.32857479770231));
#26960=CARTESIAN_POINT('Origin',(0.6,4.19441528707968E-16,6.85));
#26961=CARTESIAN_POINT('Origin',(0.6,4.19441528707968E-16,6.85));
#26962=CARTESIAN_POINT('Origin',(0.6,4.19441528707968E-16,6.85));
#26963=CARTESIAN_POINT('Origin',(0.6,2.62138151170087,6.32857479770231));
#26964=CARTESIAN_POINT('Origin',(0.6,2.62138151170087,6.32857479770231));
#26965=CARTESIAN_POINT('Origin',(0.6,2.62138151170087,6.32857479770231));
#26966=CARTESIAN_POINT('Origin',(0.6,4.84368145112785,4.84368145112785));
#26967=CARTESIAN_POINT('Origin',(0.6,4.84368145112785,4.84368145112785));
#26968=CARTESIAN_POINT('Origin',(0.6,4.84368145112785,4.84368145112785));
#26969=CARTESIAN_POINT('Origin',(0.6,6.32857479770231,2.62138151170086));
#26970=CARTESIAN_POINT('Origin',(0.6,6.32857479770231,2.62138151170086));
#26971=CARTESIAN_POINT('Origin',(0.6,6.32857479770231,2.62138151170086));
#26972=CARTESIAN_POINT('Origin',(0.6,6.85,0.));
#26973=CARTESIAN_POINT('Origin',(0.6,6.85,0.));
#26974=CARTESIAN_POINT('Origin',(0.6,6.85,0.));
#26975=CARTESIAN_POINT('Origin',(0.25,0.,0.));
#26976=CARTESIAN_POINT('',(0.25,-6.25,-7.65404249467096E-16));
#37160=UNCERTAINTY_MEASURE_WITH_UNIT(LENGTH_MEASURE(0.01),#37182,
'DISTANCE_ACCURACY_VALUE',
'Maximum model space distance between geometric entities at asserted c
onnectivities');
#37166=UNCERTAINTY_MEASURE_WITH_UNIT(LENGTH_MEASURE(0.01),#37182,
'DISTANCE_ACCURACY_VALUE',
'Maximum model space distance between geometric entities at asserted c
onnectivities');
#37175=(
GEOMETRIC_REPRESENTATION_CONTEXT(3)
GLOBAL_UNCERTAINTY_ASSIGNED_CONTEXT((#37160))
GLOBAL_UNIT_ASSIGNED_CONTEXT((#37182,#37184,#37185))
REPRESENTATION_CONTEXT('','3D')
);
#37181=(
GEOMETRIC_REPRESENTATION_CONTEXT(3)
GLOBAL_UNCERTAINTY_ASSIGNED_CONTEXT((#37166))
GLOBAL_UNIT_ASSIGNED_CONTEXT((#37182,#37184,#37185))
REPRESENTATION_CONTEXT('','3D')
);
#37182=(
LENGTH_UNIT()
NAMED_UNIT(*)
SI_UNIT(.MILLI.,.METRE.)
);
#37184=(
NAMED_UNIT(*)
PLANE_ANGLE_UNIT()
SI_UNIT($,.RADIAN.)
);
#37185=(
NAMED_UNIT(*)
SI_UNIT($,.STERADIAN.)
SOLID_ANGLE_UNIT()
);
#37194=SHAPE_DEFINITION_REPRESENTATION(#37208,#37245);
#37208=PRODUCT_DEFINITION_SHAPE('',$,#37260);
#37245=SHAPE_REPRESENTATION('',(#15705),#37175);
#37251=PRODUCT_DEFINITION_CONTEXT('part definition',#37295,'design');
#37260=PRODUCT_DEFINITION('2026-10-20-13-23-58-415',
'08_Knurled_Thumb_Knob_PLA',#37274,#37251);
#37274=PRODUCT_DEFINITION_FORMATION('',$,#37305);
#37295=APPLICATION_CONTEXT(
'Core Data for Automotive Mechanical Design Process');
#37296=PRODUCT_CONTEXT('part definition',#37295,'mechanical');
#37305=PRODUCT('2026-10-20-13-23-58-415','08_Knurled_Thumb_Knob_PLA',$,
(#37296));
#37381=COLOUR_RGB('Off White',0.89,0.88,0.83);
#37382=FILL_AREA_STYLE_COLOUR('',#37381);
#37383=FILL_AREA_STYLE('',(#37382));
#37384=SURFACE_STYLE_FILL_AREA(#37383);
#37385=SURFACE_SIDE_STYLE('',(#37384));
#37386=SURFACE_STYLE_USAGE(.BOTH.,#37385);
#37387=PRESENTATION_STYLE_ASSIGNMENT((#37386));
ENDSEC;
END-ISO-10303-21;
